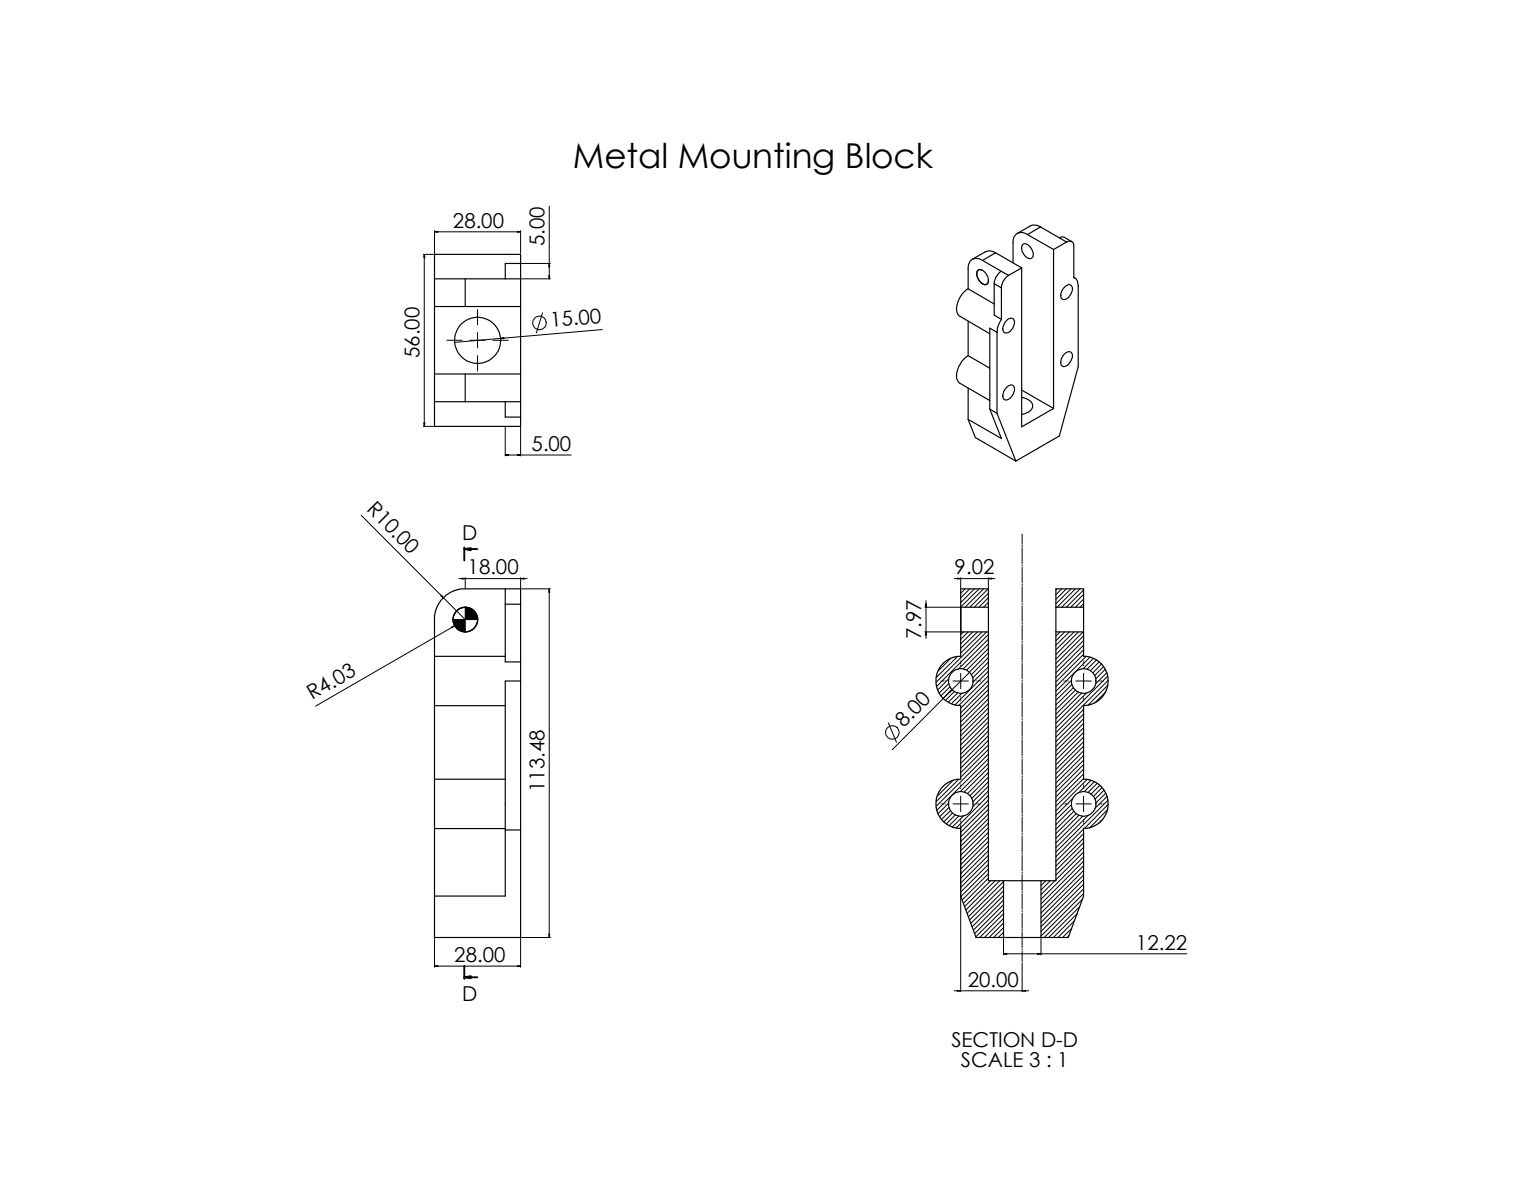
ISO-10303-21;
HEADER;
FILE_DESCRIPTION (('STEP AP214'),
    '1' );
FILE_NAME ('Metal Mounting Block.step',
    '2026-10-20T14:49:59',
    ( '' ),
    ( '' ),
    'SwSTEP 2.0',
    'SolidWorks 2025',
    '' );
FILE_SCHEMA (( 'AUTOMOTIVE_DESIGN' ));
ENDSEC;

DATA;
#3=LINE ( 'NONE', #5660, #7079 ) ;
#10=FACE_BOUND ( 'NONE', #10352, .T. ) ;
#13=VERTEX_POINT ( 'NONE', #5217 ) ;
#17=EDGE_CURVE ( 'NONE', #7054, #8863, #10257, .T. ) ;
#35=DIRECTION ( 'NONE',  ( 1.000000000000000000, -0.000000000000000000, -0.000000000000000000 ) ) ;
#39=VERTEX_POINT ( 'NONE', #5423 ) ;
#41=CARTESIAN_POINT ( 'NONE',  ( -7.293506896408097795, 145.5696653505793563, -20.00000000000000711 ) ) ;
#51=CYLINDRICAL_SURFACE ( 'NONE', #8825, 4.000000000000000000 ) ;
#52=AXIS2_PLACEMENT_3D ( 'NONE', #3037, #3895, #4040 ) ;
#61=AXIS2_PLACEMENT_3D ( 'NONE', #1587, #8044, #3822 ) ;
#66=LINE ( 'NONE', #8964, #2259 ) ;
#67=DIRECTION ( 'NONE',  ( -0.7071067811864983899, 8.659560562354331352E-17, 0.7071067811865966446 ) ) ;
#72=ORIENTED_EDGE ( 'NONE', *, *, #1454, .F. ) ;
#89=ADVANCED_FACE ( 'NONE', ( #9520 ), #9630, .T. ) ;
#91=DIRECTION ( 'NONE',  ( 0.000000000000000000, -1.222897680782651471E-16, 1.000000000000000000 ) ) ;
#95=DIRECTION ( 'NONE',  ( -0.000000000000000000, -0.000000000000000000, 1.000000000000000000 ) ) ;
#97=EDGE_LOOP ( 'NONE', ( #5379, #7947, #3762, #7012 ) ) ;
#99=ORIENTED_EDGE ( 'NONE', *, *, #5544, .F. ) ;
#104=VECTOR ( 'NONE', #4491, 1000.000000000000000 ) ;
#113=VECTOR ( 'NONE', #5634, 1000.000000000000000 ) ;
#121=VECTOR ( 'NONE', #5228, 1000.000000000000000 ) ;
#124=CIRCLE ( 'NONE', #1803, 7.500000000000000000 ) ;
#131=ORIENTED_EDGE ( 'NONE', *, *, #6804, .F. ) ;
#138=CARTESIAN_POINT ( 'NONE',  ( -7.293506896408097795, 50.54838324668256888, 20.00000000000001776 ) ) ;
#152=FACE_OUTER_BOUND ( 'NONE', #4686, .T. ) ;
#153=DIRECTION ( 'NONE',  ( -1.000000000000000000, 0.000000000000000000, 0.000000000000000000 ) ) ;
#156=ORIENTED_EDGE ( 'NONE', *, *, #9691, .F. ) ;
#157=CARTESIAN_POINT ( 'NONE',  ( -2.293506896408097795, 120.5696653505793705, 20.00000000000000711 ) ) ;
#167=ORIENTED_EDGE ( 'NONE', *, *, #1641, .F. ) ;
#188=CARTESIAN_POINT ( 'NONE',  ( -30.29350689640809335, 37.08684478514406635, 0.000000000000000000 ) ) ;
#190=CARTESIAN_POINT ( 'NONE',  ( -7.293506896408097795, 50.54838324668256888, -20.00000000000001776 ) ) ;
#195=VERTEX_POINT ( 'NONE', #3902 ) ;
#200=DIRECTION ( 'NONE',  ( 0.000000000000000000, 1.000000000000000000, 0.000000000000000000 ) ) ;
#203=EDGE_LOOP ( 'NONE', ( #8240, #8305, #10001, #6976, #3187, #9611 ) ) ;
#209=FACE_OUTER_BOUND ( 'NONE', #8382, .T. ) ;
#224=CARTESIAN_POINT ( 'NONE',  ( -30.29350689640809335, 80.56966535057935630, -24.00000000000000711 ) ) ;
#255=AXIS2_PLACEMENT_3D ( 'NONE', #5974, #6135, #9270 ) ;
#270=LINE ( 'NONE', #5923, #8481 ) ;
#272=ORIENTED_EDGE ( 'NONE', *, *, #9010, .T. ) ;
#279=FACE_OUTER_BOUND ( 'NONE', #7883, .T. ) ;
#283=EDGE_LOOP ( 'NONE', ( #4736, #4335, #5874, #8256, #8188 ) ) ;
#288=VERTEX_POINT ( 'NONE', #1021 ) ;
#295=VECTOR ( 'NONE', #753, 1000.000000000000114 ) ;
#302=EDGE_CURVE ( 'NONE', #5556, #3604, #5045, .T. ) ;
#303=EDGE_CURVE ( 'NONE', #4587, #5189, #10304, .T. ) ;
#316=VECTOR ( 'NONE', #2440, 1000.000000000000000 ) ;
#317=EDGE_CURVE ( 'NONE', #10264, #2451, #2832, .T. ) ;
#339=ORIENTED_EDGE ( 'NONE', *, *, #9708, .F. ) ;
#344=DIRECTION ( 'NONE',  ( 1.000000000000000000, -0.000000000000000000, -0.000000000000000000 ) ) ;
#353=CYLINDRICAL_SURFACE ( 'NONE', #7185, 4.000000000000000000 ) ;
#355=CYLINDRICAL_SURFACE ( 'NONE', #5843, 4.000000000000000000 ) ;
#356=EDGE_CURVE ( 'NONE', #5466, #9263, #915, .T. ) ;
#372=CARTESIAN_POINT ( 'NONE',  ( -20.29350689640809691, 140.5696653505793563, 20.00000000000002132 ) ) ;
#376=AXIS2_PLACEMENT_3D ( 'NONE', #9836, #6639, #8122 ) ;
#383=ORIENTED_EDGE ( 'NONE', *, *, #664, .T. ) ;
#398=DIRECTION ( 'NONE',  ( 1.000000000000000000, -0.000000000000000000, -0.000000000000000000 ) ) ;
#410=EDGE_LOOP ( 'NONE', ( #1681, #5239, #2854, #5762 ) ) ;
#418=CARTESIAN_POINT ( 'NONE',  ( -7.293506896408097795, 4.007378841484243628E-15, -28.00000000000002132 ) ) ;
#419=ORIENTED_EDGE ( 'NONE', *, *, #2627, .T. ) ;
#432=DIRECTION ( 'NONE',  ( 1.000000000000000000, -0.000000000000000000, -0.000000000000000000 ) ) ;
#438=ORIENTED_EDGE ( 'NONE', *, *, #7577, .T. ) ;
#443=ORIENTED_EDGE ( 'NONE', *, *, #6054, .F. ) ;
#450=ORIENTED_EDGE ( 'NONE', *, *, #5738, .F. ) ;
#452=VECTOR ( 'NONE', #3941, 1000.000000000000000 ) ;
#458=DIRECTION ( 'NONE',  ( 0.000000000000000000, 0.000000000000000000, 1.000000000000000000 ) ) ;
#467=VECTOR ( 'NONE', #4578, 1000.000000000000114 ) ;
#469=DIRECTION ( 'NONE',  ( 1.000000000000000000, 0.000000000000000000, 0.000000000000000000 ) ) ;
#476=VECTOR ( 'NONE', #3446, 1000.000000000000000 ) ;
#484=DIRECTION ( 'NONE',  ( 0.000000000000000000, -1.000000000000000000, 1.222897680782651471E-16 ) ) ;
#489=ADVANCED_FACE ( 'NONE', ( #10089 ), #9183, .T. ) ;
#495=DIRECTION ( 'NONE',  ( 0.000000000000000000, -1.000000000000000000, -1.222897680782651224E-16 ) ) ;
#504=DIRECTION ( 'NONE',  ( 1.000000000000000000, 0.000000000000000000, 0.000000000000000000 ) ) ;
#510=VERTEX_POINT ( 'NONE', #5251 ) ;
#512=ORIENTED_EDGE ( 'NONE', *, *, #1198, .F. ) ;
#522=DIRECTION ( 'NONE',  ( -1.000000000000000000, -0.000000000000000000, -0.000000000000000000 ) ) ;
#524=CARTESIAN_POINT ( 'NONE',  ( -30.29350689640809335, 140.5696653505793563, -20.00000000000000355 ) ) ;
#544=CARTESIAN_POINT ( 'NONE',  ( -30.29350689640809335, 37.08684478514406635, -15.00000000000000355 ) ) ;
#545=ADVANCED_FACE ( 'NONE', ( #7912, #2343, #6211, #4819, #2293 ), #3832, .F. ) ;
#567=ORIENTED_EDGE ( 'NONE', *, *, #7866, .T. ) ;
#579=CARTESIAN_POINT ( 'NONE',  ( -20.29350689640809691, 140.5696653505793563, -20.00000000000000355 ) ) ;
#582=CIRCLE ( 'NONE', #8191, 5.000000000000000888 ) ;
#592=ORIENTED_EDGE ( 'NONE', *, *, #303, .F. ) ;
#596=VERTEX_POINT ( 'NONE', #7217 ) ;
#603=ORIENTED_EDGE ( 'NONE', *, *, #3823, .F. ) ;
#621=CARTESIAN_POINT ( 'NONE',  ( -30.29350689640809335, 145.5696653505793563, 20.00000000000000711 ) ) ;
#633=DIRECTION ( 'NONE',  ( 0.000000000000000000, -1.000000000000000000, 0.000000000000000000 ) ) ;
#634=EDGE_CURVE ( 'NONE', #2019, #13, #4708, .T. ) ;
#656=PLANE ( 'NONE',  #8662 ) ;
#657=CARTESIAN_POINT ( 'NONE',  ( -7.293506896408097795, 4.007378841484243628E-15, 28.00000000000002132 ) ) ;
#658=CARTESIAN_POINT ( 'NONE',  ( -7.293506896408097795, 80.56966535057935630, -20.00000000000000711 ) ) ;
#660=CIRCLE ( 'NONE', #4540, 4.000000000000000000 ) ;
#664=EDGE_CURVE ( 'NONE', #954, #4361, #955, .T. ) ;
#667=DIRECTION ( 'NONE',  ( 0.000000000000000000, 0.000000000000000000, 1.000000000000000000 ) ) ;
#675=EDGE_LOOP ( 'NONE', ( #1333, #9999, #2381, #686 ) ) ;
#676=ADVANCED_FACE ( 'NONE', ( #10, #4242 ), #5668, .F. ) ;
#686=ORIENTED_EDGE ( 'NONE', *, *, #10087, .F. ) ;
#716=VERTEX_POINT ( 'NONE', #2543 ) ;
#731=EDGE_CURVE ( 'NONE', #8244, #5058, #3289, .T. ) ;
#734=CIRCLE ( 'NONE', #7849, 4.000000000000000000 ) ;
#737=DIRECTION ( 'NONE',  ( 0.000000000000000000, 0.000000000000000000, 1.000000000000000000 ) ) ;
#740=CARTESIAN_POINT ( 'NONE',  ( -7.293506896408097795, 145.5696653505793563, -25.00000000000000711 ) ) ;
#750=AXIS2_PLACEMENT_3D ( 'NONE', #8663, #6275, #5427 ) ;
#753=DIRECTION ( 'NONE',  ( 0.000000000000000000, -0.9374252720097652203, -0.3481865296036273372 ) ) ;
#761=CARTESIAN_POINT ( 'NONE',  ( -7.293506896408097795, 80.56966535057935630, 20.00000000000000711 ) ) ;
#763=AXIS2_PLACEMENT_3D ( 'NONE', #4850, #200, #3320 ) ;
#767=DIRECTION ( 'NONE',  ( -1.000000000000000000, 0.000000000000000000, 0.000000000000000000 ) ) ;
#777=LINE ( 'NONE', #4799, #5594 ) ;
#780=VECTOR ( 'NONE', #9895, 1000.000000000000000 ) ;
#781=EDGE_LOOP ( 'NONE', ( #592, #10254 ) ) ;
#782=DIRECTION ( 'NONE',  ( 1.000000000000000000, -0.000000000000000000, -0.000000000000000000 ) ) ;
#793=CIRCLE ( 'NONE', #2484, 3.999999999999989786 ) ;
#801=DIRECTION ( 'NONE',  ( 0.000000000000000000, -1.000000000000000000, -1.222897680782651471E-16 ) ) ;
#812=ORIENTED_EDGE ( 'NONE', *, *, #634, .T. ) ;
#822=VERTEX_POINT ( 'NONE', #4455 ) ;
#827=DIRECTION ( 'NONE',  ( 0.000000000000000000, 0.000000000000000000, 1.000000000000000000 ) ) ;
#832=VECTOR ( 'NONE', #8468, 1000.000000000000000 ) ;
#843=ORIENTED_EDGE ( 'NONE', *, *, #5371, .T. ) ;
#846=EDGE_CURVE ( 'NONE', #10164, #6362, #660, .T. ) ;
#848=DIRECTION ( 'NONE',  ( 1.000000000000000000, 0.000000000000000000, -0.000000000000000000 ) ) ;
#850=DIRECTION ( 'NONE',  ( 0.000000000000000000, -1.734723475976808278E-15, 1.000000000000000000 ) ) ;
#852=VERTEX_POINT ( 'NONE', #2061 ) ;
#855=DIRECTION ( 'NONE',  ( 0.000000000000000000, -0.9374252720097652203, 0.3481865296036273372 ) ) ;
#856=EDGE_CURVE ( 'NONE', #6933, #6085, #6838, .T. ) ;
#859=AXIS2_PLACEMENT_3D ( 'NONE', #9746, #8298, #5696 ) ;
#860=CARTESIAN_POINT ( 'NONE',  ( -20.29350689640809691, 150.5696653505793563, 20.00000000000000355 ) ) ;
#861=DIRECTION ( 'NONE',  ( 0.000000000000000000, -1.000000000000000000, -1.222897680782651224E-16 ) ) ;
#875=ORIENTED_EDGE ( 'NONE', *, *, #5133, .T. ) ;
#878=DIRECTION ( 'NONE',  ( 0.000000000000000000, -1.000000000000000000, 0.000000000000000000 ) ) ;
#885=CARTESIAN_POINT ( 'NONE',  ( -30.29350689640809335, -0.3998014571812398832, 1.076388538564875708 ) ) ;
#904=DIRECTION ( 'NONE',  ( 1.000000000000000000, -0.000000000000000000, -0.000000000000000000 ) ) ;
#911=DIRECTION ( 'NONE',  ( 0.000000000000000000, 0.000000000000000000, 1.000000000000000000 ) ) ;
#915=LINE ( 'NONE', #4150, #9967 ) ;
#931=CARTESIAN_POINT ( 'NONE',  ( -16.29350689640809691, -19.43033464942062238, 0.000000000000000000 ) ) ;
#935=CARTESIAN_POINT ( 'NONE',  ( -20.29350689640809691, 140.5696653505793563, -20.00000000000000711 ) ) ;
#938=DIRECTION ( 'NONE',  ( 1.000000000000000000, -0.000000000000000000, -0.000000000000000000 ) ) ;
#941=VERTEX_POINT ( 'NONE', #3973 ) ;
#942=DIRECTION ( 'NONE',  ( -1.000000000000000000, -0.000000000000000000, -0.000000000000000000 ) ) ;
#945=LINE ( 'NONE', #2479, #10150 ) ;
#946=DIRECTION ( 'NONE',  ( 0.000000000000000000, -0.9374252720097652203, 0.3481865296036273372 ) ) ;
#952=ORIENTED_EDGE ( 'NONE', *, *, #17, .F. ) ;
#954=VERTEX_POINT ( 'NONE', #10390 ) ;
#955=LINE ( 'NONE', #8910, #476 ) ;
#966=ORIENTED_EDGE ( 'NONE', *, *, #993, .T. ) ;
#992=DIRECTION ( 'NONE',  ( -1.000000000000000000, 0.000000000000000000, 0.000000000000000000 ) ) ;
#993=EDGE_CURVE ( 'NONE', #2923, #9336, #1538, .T. ) ;
#1003=( GEOMETRIC_REPRESENTATION_CONTEXT ( 3 ) GLOBAL_UNCERTAINTY_ASSIGNED_CONTEXT ( ( #1512 ) ) GLOBAL_UNIT_ASSIGNED_CONTEXT ( ( #2813, #9988, #8280 ) ) REPRESENTATION_CONTEXT ( 'NONE', 'WORKASPACE' ) );
#1006=EDGE_CURVE ( 'NONE', #6072, #6663, #8634, .T. ) ;
#1015=LINE ( 'NONE', #524, #8409 ) ;
#1020=PRODUCT_DEFINITION_CONTEXT ( 'detailed design', #8151, 'design' ) ;
#1021=CARTESIAN_POINT ( 'NONE',  ( -16.29350689640810756, 140.5696653505793563, -10.98204862120179648 ) ) ;
#1034=VECTOR ( 'NONE', #1710, 1000.000000000000000 ) ;
#1036=FACE_OUTER_BOUND ( 'NONE', #9629, .T. ) ;
#1043=VERTEX_POINT ( 'NONE', #1377 ) ;
#1049=VECTOR ( 'NONE', #861, 1000.000000000000000 ) ;
#1060=LINE ( 'NONE', #6623, #5109 ) ;
#1069=ORIENTED_EDGE ( 'NONE', *, *, #8198, .T. ) ;
#1071=ORIENTED_EDGE ( 'NONE', *, *, #664, .F. ) ;
#1074=LINE ( 'NONE', #1819, #4670 ) ;
#1079=VERTEX_POINT ( 'NONE', #5656 ) ;
#1080=LINE ( 'NONE', #1926, #7329 ) ;
#1083=VERTEX_POINT ( 'NONE', #8893 ) ;
#1088=DIRECTION ( 'NONE',  ( 1.000000000000000000, -0.000000000000000000, -0.000000000000000000 ) ) ;
#1100=ORIENTED_EDGE ( 'NONE', *, *, #4696, .T. ) ;
#1101=CARTESIAN_POINT ( 'NONE',  ( -2.293506896408097795, 145.5696653505793563, -25.00000000000000711 ) ) ;
#1102=DIRECTION ( 'NONE',  ( 1.000000000000000000, 0.000000000000000000, 0.000000000000000000 ) ) ;
#1105=CARTESIAN_POINT ( 'NONE',  ( -20.29350689640809691, 140.5696653505793563, 0.000000000000000000 ) ) ;
#1109=ORIENTED_EDGE ( 'NONE', *, *, #3823, .T. ) ;
#1111=DIRECTION ( 'NONE',  ( -1.000000000000000000, 0.000000000000000000, 0.000000000000000000 ) ) ;
#1116=LINE ( 'NONE', #7323, #6386 ) ;
#1117=VERTEX_POINT ( 'NONE', #7257 ) ;
#1131=CIRCLE ( 'NONE', #7064, 10.00000000000000888 ) ;
#1140=EDGE_CURVE ( 'NONE', #10264, #9816, #2426, .T. ) ;
#1142=CARTESIAN_POINT ( 'NONE',  ( -30.29350689640809335, 80.56966535057935630, 20.00000000000000711 ) ) ;
#1146=EDGE_LOOP ( 'NONE', ( #812, #8947 ) ) ;
#1148=CARTESIAN_POINT ( 'NONE',  ( -20.29350689640809691, 140.5696653505793563, 20.00000000000000355 ) ) ;
#1152=CIRCLE ( 'NONE', #3873, 4.000000000000000000 ) ;
#1157=CARTESIAN_POINT ( 'NONE',  ( -30.29350689640809335, 37.08684478514406635, 15.00000000000000355 ) ) ;
#1160=FACE_OUTER_BOUND ( 'NONE', #2223, .T. ) ;
#1161=VECTOR ( 'NONE', #7788, 1000.000000000000000 ) ;
#1167=ORIENTED_EDGE ( 'NONE', *, *, #8133, .T. ) ;
#1175=EDGE_LOOP ( 'NONE', ( #6473, #7794, #10471, #9288 ) ) ;
#1183=DIRECTION ( 'NONE',  ( -1.000000000000000000, 0.000000000000000000, 0.000000000000000000 ) ) ;
#1190=DIRECTION ( 'NONE',  ( 0.000000000000000000, 0.000000000000000000, 1.000000000000000000 ) ) ;
#1193=FACE_OUTER_BOUND ( 'NONE', #1279, .T. ) ;
#1196=ORIENTED_EDGE ( 'NONE', *, *, #1532, .F. ) ;
#1198=EDGE_CURVE ( 'NONE', #5466, #7089, #3190, .T. ) ;
#1199=EDGE_CURVE ( 'NONE', #5863, #1913, #1792, .T. ) ;
#1205=ORIENTED_EDGE ( 'NONE', *, *, #2933, .T. ) ;
#1206=DIRECTION ( 'NONE',  ( 0.000000000000000000, -1.000000000000000000, -1.222897680782651224E-16 ) ) ;
#1220=EDGE_CURVE ( 'NONE', #4525, #2500, #3708, .T. ) ;
#1225=CARTESIAN_POINT ( 'NONE',  ( -2.293506896408097795, 150.5696653505793563, 20.00000000000000711 ) ) ;
#1234=DIRECTION ( 'NONE',  ( 0.000000000000000000, -1.431206729101514631E-16, 1.000000000000000000 ) ) ;
#1247=VECTOR ( 'NONE', #1264, 1000.000000000000000 ) ;
#1249=ORIENTED_EDGE ( 'NONE', *, *, #7540, .T. ) ;
#1258=LINE ( 'NONE', #2847, #104 ) ;
#1264=DIRECTION ( 'NONE',  ( 1.000000000000000000, -0.000000000000000000, -0.000000000000000000 ) ) ;
#1265=PLANE ( 'NONE',  #6164 ) ;
#1268=EDGE_LOOP ( 'NONE', ( #3343, #2802, #567, #512, #4602, #10138, #10269 ) ) ;
#1276=DIRECTION ( 'NONE',  ( 1.000000000000000000, -0.000000000000000000, -0.000000000000000000 ) ) ;
#1279=EDGE_LOOP ( 'NONE', ( #3702, #9720, #2445, #3175 ) ) ;
#1282=VERTEX_POINT ( 'NONE', #9970 ) ;
#1291=EDGE_LOOP ( 'NONE', ( #7966, #7553 ) ) ;
#1295=ORIENTED_EDGE ( 'NONE', *, *, #7737, .F. ) ;
#1302=DIRECTION ( 'NONE',  ( 1.000000000000000000, -0.000000000000000000, -0.000000000000000000 ) ) ;
#1311=ORIENTED_EDGE ( 'NONE', *, *, #2487, .F. ) ;
#1312=LINE ( 'NONE', #7938, #10266 ) ;
#1315=CARTESIAN_POINT ( 'NONE',  ( -30.29350689640809335, 120.5696653505793705, -20.00000000000000711 ) ) ;
#1318=FACE_OUTER_BOUND ( 'NONE', #283, .T. ) ;
#1322=EDGE_CURVE ( 'NONE', #10164, #4525, #1258, .T. ) ;
#1331=DIRECTION ( 'NONE',  ( 0.000000000000000000, 0.000000000000000000, 1.000000000000000000 ) ) ;
#1333=ORIENTED_EDGE ( 'NONE', *, *, #9472, .T. ) ;
#1334=ORIENTED_EDGE ( 'NONE', *, *, #1987, .T. ) ;
#1339=ORIENTED_EDGE ( 'NONE', *, *, #1006, .F. ) ;
#1340=VECTOR ( 'NONE', #10000, 1000.000000000000000 ) ;
#1344=CYLINDRICAL_SURFACE ( 'NONE', #2810, 3.999999999999989786 ) ;
#1352=VERTEX_POINT ( 'NONE', #8306 ) ;
#1353=EDGE_CURVE ( 'NONE', #9176, #941, #4338, .T. ) ;
#1354=CARTESIAN_POINT ( 'NONE',  ( -7.293506896408097795, 126.8146633489777599, 25.00000000000000355 ) ) ;
#1359=VERTEX_POINT ( 'NONE', #1101 ) ;
#1367=EDGE_LOOP ( 'NONE', ( #7375, #167, #6674, #5877 ) ) ;
#1370=CARTESIAN_POINT ( 'NONE',  ( -16.26850689640809478, 140.5696653505793563, 20.00000000000002132 ) ) ;
#1377=CARTESIAN_POINT ( 'NONE',  ( -16.29350689640809691, 55.56966535057936341, -7.500000000000000000 ) ) ;
#1380=EDGE_CURVE ( 'NONE', #8244, #9480, #7671, .T. ) ;
#1403=VERTEX_POINT ( 'NONE', #3862 ) ;
#1405=CIRCLE ( 'NONE', #52, 5.000000000000000888 ) ;
#1407=ADVANCED_FACE ( 'NONE', ( #3750 ), #2157, .T. ) ;
#1418=ORIENTED_EDGE ( 'NONE', *, *, #9964, .T. ) ;
#1419=DIRECTION ( 'NONE',  ( 1.000000000000000000, 0.000000000000000000, 0.000000000000000000 ) ) ;
#1439=VERTEX_POINT ( 'NONE', #8785 ) ;
#1442=ORIENTED_EDGE ( 'NONE', *, *, #5543, .T. ) ;
#1454=EDGE_CURVE ( 'NONE', #5461, #6490, #1312, .T. ) ;
#1468=ADVANCED_FACE ( 'NONE', ( #1526 ), #3056, .T. ) ;
#1471=DIRECTION ( 'NONE',  ( -1.000000000000000000, 0.000000000000000000, 0.000000000000000000 ) ) ;
#1481=DIRECTION ( 'NONE',  ( -0.000000000000000000, 1.222897680782651471E-16, -1.000000000000000000 ) ) ;
#1485=VECTOR ( 'NONE', #3097, 1000.000000000000000 ) ;
#1501=AXIS2_PLACEMENT_3D ( 'NONE', #5590, #8724, #1471 ) ;
#1512=UNCERTAINTY_MEASURE_WITH_UNIT (LENGTH_MEASURE( 1.000000000000000082E-05 ), #2813, 'distance_accuracy_value', 'NONE');
#1516=EDGE_CURVE ( 'NONE', #2007, #1282, #9590, .T. ) ;
#1526=FACE_OUTER_BOUND ( 'NONE', #1367, .T. ) ;
#1532=EDGE_CURVE ( 'NONE', #9083, #1931, #1954, .T. ) ;
#1537=ORIENTED_EDGE ( 'NONE', *, *, #7658, .T. ) ;
#1538=LINE ( 'NONE', #5561, #7759 ) ;
#1541=LINE ( 'NONE', #3975, #3278 ) ;
#1546=VECTOR ( 'NONE', #3114, 1000.000000000000000 ) ;
#1552=AXIS2_PLACEMENT_3D ( 'NONE', #7863, #7967, #10359 ) ;
#1556=ORIENTED_EDGE ( 'NONE', *, *, #6748, .F. ) ;
#1571=ORIENTED_EDGE ( 'NONE', *, *, #634, .F. ) ;
#1587=CARTESIAN_POINT ( 'NONE',  ( -30.29350689640809335, 80.56966535057935630, -20.00000000000000711 ) ) ;
#1593=ORIENTED_EDGE ( 'NONE', *, *, #4957, .F. ) ;
#1594=EDGE_CURVE ( 'NONE', #5925, #3441, #1074, .T. ) ;
#1596=LINE ( 'NONE', #8757, #5448 ) ;
#1597=AXIS2_PLACEMENT_3D ( 'NONE', #5049, #7006, #484 ) ;
#1624=CARTESIAN_POINT ( 'NONE',  ( -7.293506896408097795, -3.651280424770854409E-15, 24.99999999999998579 ) ) ;
#1632=EDGE_LOOP ( 'NONE', ( #2607, #2789, #4830, #9276, #8779, #2786, #443, #7436, #10424, #10141, #9748, #952, #4956, #10358, #2505, #2868, #10031, #8560, #156, #3347 ) ) ;
#1633=DIRECTION ( 'NONE',  ( 0.000000000000000000, 0.000000000000000000, 1.000000000000000000 ) ) ;
#1637=LINE ( 'NONE', #1796, #4788 ) ;
#1641=EDGE_CURVE ( 'NONE', #1403, #5730, #6745, .T. ) ;
#1653=ORIENTED_EDGE ( 'NONE', *, *, #1641, .T. ) ;
#1654=ADVANCED_FACE ( 'NONE', ( #1920 ), #3363, .F. ) ;
#1668=LINE ( 'NONE', #188, #113 ) ;
#1669=EDGE_CURVE ( 'NONE', #2192, #195, #5789, .T. ) ;
#1676=DIRECTION ( 'NONE',  ( -1.000000000000000000, 0.000000000000000000, 0.000000000000000000 ) ) ;
#1681=ORIENTED_EDGE ( 'NONE', *, *, #846, .T. ) ;
#1682=DIRECTION ( 'NONE',  ( -1.000000000000000000, 0.000000000000000000, 0.000000000000000000 ) ) ;
#1683=EDGE_CURVE ( 'NONE', #1083, #1913, #4521, .T. ) ;
#1686=DIRECTION ( 'NONE',  ( 0.000000000000000000, 1.000000000000000000, -1.460512169908342690E-16 ) ) ;
#1691=CARTESIAN_POINT ( 'NONE',  ( -7.293506896408105789, 150.5696653505793563, -20.00000000000000355 ) ) ;
#1695=VERTEX_POINT ( 'NONE', #7756 ) ;
#1706=CIRCLE ( 'NONE', #8135, 7.999999999999991118 ) ;
#1710=DIRECTION ( 'NONE',  ( -0.000000000000000000, -0.000000000000000000, 1.000000000000000000 ) ) ;
#1719=VECTOR ( 'NONE', #6591, 1000.000000000000000 ) ;
#1728=DIRECTION ( 'NONE',  ( -1.000000000000000000, 0.000000000000000000, 0.000000000000000000 ) ) ;
#1734=AXIS2_PLACEMENT_3D ( 'NONE', #8821, #10265, #8024 ) ;
#1736=CARTESIAN_POINT ( 'NONE',  ( -30.29350689640809335, -0.3998014571812398832, -1.076388538564875708 ) ) ;
#1744=CARTESIAN_POINT ( 'NONE',  ( -20.29350689640810401, 150.5696653505793563, -10.98204862120179826 ) ) ;
#1748=AXIS2_PLACEMENT_3D ( 'NONE', #3396, #6681, #1860 ) ;
#1762=UNCERTAINTY_MEASURE_WITH_UNIT (LENGTH_MEASURE( 1.000000000000000082E-05 ), #9279, 'distance_accuracy_value', 'NONE');
#1772=EDGE_CURVE ( 'NONE', #510, #4261, #8231, .T. ) ;
#1773=ADVANCED_FACE ( 'NONE', ( #8650 ), #1344, .F. ) ;
#1776=ORIENTED_EDGE ( 'NONE', *, *, #6748, .T. ) ;
#1784=FACE_OUTER_BOUND ( 'NONE', #6548, .T. ) ;
#1786=EDGE_CURVE ( 'NONE', #954, #9488, #2649, .T. ) ;
#1788=EDGE_LOOP ( 'NONE', ( #8956, #7525, #5665, #603 ) ) ;
#1792=LINE ( 'NONE', #4859, #8780 ) ;
#1793=CARTESIAN_POINT ( 'NONE',  ( -7.293506896408097795, -3.651280424770854409E-15, -24.99999999999998579 ) ) ;
#1796=CARTESIAN_POINT ( 'NONE',  ( -7.293506896408097795, 72.08684478514406635, 28.00000000000001066 ) ) ;
#1803=AXIS2_PLACEMENT_3D ( 'NONE', #5143, #9067, #3562 ) ;
#1804=ORIENTED_EDGE ( 'NONE', *, *, #7866, .F. ) ;
#1814=AXIS2_PLACEMENT_3D ( 'NONE', #1142, #1088, #6757 ) ;
#1819=CARTESIAN_POINT ( 'NONE',  ( -7.293506896408097795, 2.445795361565304815E-15, -20.00000000000002132 ) ) ;
#1831=EDGE_CURVE ( 'NONE', #4261, #596, #7858, .T. ) ;
#1837=AXIS2_PLACEMENT_3D ( 'NONE', #5705, #6667, #1633 ) ;
#1838=ORIENTED_EDGE ( 'NONE', *, *, #2430, .T. ) ;
#1844=CARTESIAN_POINT ( 'NONE',  ( -30.29350689640809335, 50.54838324668256888, 20.00000000000001776 ) ) ;
#1845=ADVANCED_FACE ( 'NONE', ( #4726 ), #8704, .F. ) ;
#1860=DIRECTION ( 'NONE',  ( 0.000000000000000000, 0.000000000000000000, 1.000000000000000000 ) ) ;
#1861=CYLINDRICAL_SURFACE ( 'NONE', #8080, 4.000000000000000000 ) ;
#1870=CARTESIAN_POINT ( 'NONE',  ( -2.293506896408097795, 145.5696653505793563, 20.00000000000000711 ) ) ;
#1871=CARTESIAN_POINT ( 'NONE',  ( -24.29350689640808980, 140.5696653505793563, 19.97500000000000853 ) ) ;
#1888=EDGE_CURVE ( 'NONE', #822, #7959, #6023, .T. ) ;
#1891=ORIENTED_EDGE ( 'NONE', *, *, #856, .T. ) ;
#1894=DIRECTION ( 'NONE',  ( -1.000000000000000000, 0.000000000000000000, 0.000000000000000000 ) ) ;
#1897=VECTOR ( 'NONE', #9971, 1000.000000000000000 ) ;
#1898=DIRECTION ( 'NONE',  ( 1.000000000000000000, 0.000000000000000000, 0.000000000000000000 ) ) ;
#1911=FACE_OUTER_BOUND ( 'NONE', #1175, .T. ) ;
#1913=VERTEX_POINT ( 'NONE', #7172 ) ;
#1920=FACE_OUTER_BOUND ( 'NONE', #3172, .T. ) ;
#1926=CARTESIAN_POINT ( 'NONE',  ( -30.29350689640809335, 120.5696653505793705, 16.00000000000000711 ) ) ;
#1931=VERTEX_POINT ( 'NONE', #5291 ) ;
#1937=DIRECTION ( 'NONE',  ( 0.000000000000000000, 0.000000000000000000, 1.000000000000000000 ) ) ;
#1942=PLANE ( 'NONE',  #7568 ) ;
#1948=DIRECTION ( 'NONE',  ( 1.000000000000000000, -0.000000000000000000, -0.000000000000000000 ) ) ;
#1954=CIRCLE ( 'NONE', #8733, 3.999999999999989786 ) ;
#1956=( NAMED_UNIT ( * ) PLANE_ANGLE_UNIT ( ) SI_UNIT ( $, .RADIAN. ) );
#1971=DIRECTION ( 'NONE',  ( -1.000000000000000000, 0.000000000000000000, 0.000000000000000000 ) ) ;
#1981=AXIS2_PLACEMENT_3D ( 'NONE', #1736, #2735, #4229 ) ;
#1983=DIRECTION ( 'NONE',  ( 1.000000000000000000, -0.000000000000000000, -0.000000000000000000 ) ) ;
#1987=EDGE_CURVE ( 'NONE', #5429, #6933, #4007, .T. ) ;
#1993=CARTESIAN_POINT ( 'NONE',  ( -30.29350689640809335, 128.5696653505793847, 20.00000000000000711 ) ) ;
#1998=LINE ( 'NONE', #7037, #7228 ) ;
#2004=DIRECTION ( 'NONE',  ( -1.000000000000000000, 0.000000000000000000, 0.000000000000000000 ) ) ;
#2007=VERTEX_POINT ( 'NONE', #10178 ) ;
#2019=VERTEX_POINT ( 'NONE', #2910 ) ;
#2026=DIRECTION ( 'NONE',  ( 0.000000000000000000, 1.000000000000000000, 1.460512169908342690E-16 ) ) ;
#2027=DIRECTION ( 'NONE',  ( -1.000000000000000000, 0.000000000000000000, 0.000000000000000000 ) ) ;
#2035=CARTESIAN_POINT ( 'NONE',  ( -30.29350689640809335, -0.3998014571812398832, 1.076388538564875708 ) ) ;
#2043=ORIENTED_EDGE ( 'NONE', *, *, #1322, .T. ) ;
#2055=CIRCLE ( 'NONE', #9857, 7.999999999999991118 ) ;
#2058=ORIENTED_EDGE ( 'NONE', *, *, #1831, .F. ) ;
#2061=CARTESIAN_POINT ( 'NONE',  ( -30.29350689640809335, 140.5696653505793563, -20.00000000000000355 ) ) ;
#2062=LINE ( 'NONE', #4456, #8497 ) ;
#2067=CARTESIAN_POINT ( 'NONE',  ( -30.29350689640809335, 120.5696653505793705, 20.00000000000000711 ) ) ;
#2097=ORIENTED_EDGE ( 'NONE', *, *, #3900, .F. ) ;
#2103=DIRECTION ( 'NONE',  ( 0.000000000000000000, 0.000000000000000000, 1.000000000000000000 ) ) ;
#2107=LINE ( 'NONE', #10065, #4468 ) ;
#2109=ADVANCED_FACE ( 'NONE', ( #4712 ), #8093, .T. ) ;
#2116=AXIS2_PLACEMENT_3D ( 'NONE', #8691, #10346, #3824 ) ;
#2121=EDGE_CURVE ( 'NONE', #6484, #6663, #2373, .T. ) ;
#2125=EDGE_CURVE ( 'NONE', #9816, #288, #793, .T. ) ;
#2127=ORIENTED_EDGE ( 'NONE', *, *, #5471, .T. ) ;
#2145=CIRCLE ( 'NONE', #2819, 4.000000000000000000 ) ;
#2149=ORIENTED_EDGE ( 'NONE', *, *, #7672, .F. ) ;
#2157=CYLINDRICAL_SURFACE ( 'NONE', #3488, 5.000000000000000888 ) ;
#2158=LINE ( 'NONE', #8124, #1049 ) ;
#2173=ORIENTED_EDGE ( 'NONE', *, *, #8842, .T. ) ;
#2180=AXIS2_PLACEMENT_3D ( 'NONE', #5276, #767, #7880 ) ;
#2189=DIRECTION ( 'NONE',  ( 0.000000000000000000, 0.000000000000000000, 1.000000000000000000 ) ) ;
#2192=VERTEX_POINT ( 'NONE', #8040 ) ;
#2201=DIRECTION ( 'NONE',  ( -1.000000000000000000, 0.000000000000000000, 0.000000000000000000 ) ) ;
#2206=EDGE_LOOP ( 'NONE', ( #2312, #10473, #7213, #131 ) ) ;
#2218=PRODUCT_DEFINITION_SHAPE ( 'NONE', 'NONE',  #6773 ) ;
#2219=EDGE_CURVE ( 'NONE', #288, #9816, #5526, .T. ) ;
#2223=EDGE_LOOP ( 'NONE', ( #3669, #9856, #2555, #8359 ) ) ;
#2230=CARTESIAN_POINT ( 'NONE',  ( -20.29350689640809691, 140.5696653505793563, 20.00000000000002132 ) ) ;
#2235=ADVANCED_FACE ( 'NONE', ( #5810 ), #7567, .F. ) ;
#2238=EDGE_LOOP ( 'NONE', ( #3655, #6176 ) ) ;
#2244=FACE_OUTER_BOUND ( 'NONE', #5322, .T. ) ;
#2245=EDGE_CURVE ( 'NONE', #1079, #7959, #5067, .T. ) ;
#2257=ORIENTED_EDGE ( 'NONE', *, *, #5471, .F. ) ;
#2259=VECTOR ( 'NONE', #9983, 1000.000000000000000 ) ;
#2262=CARTESIAN_POINT ( 'NONE',  ( -7.293506896408097795, 80.56966535057935630, -20.00000000000000711 ) ) ;
#2274=LINE ( 'NONE', #8789, #5355 ) ;
#2290=ORIENTED_EDGE ( 'NONE', *, *, #302, .F. ) ;
#2292=ADVANCED_FACE ( 'NONE', ( #5913 ), #1942, .T. ) ;
#2293=FACE_BOUND ( 'NONE', #2238, .T. ) ;
#2306=EDGE_CURVE ( 'NONE', #4058, #5577, #2145, .T. ) ;
#2312=ORIENTED_EDGE ( 'NONE', *, *, #317, .F. ) ;
#2343=FACE_BOUND ( 'NONE', #1146, .T. ) ;
#2352=VECTOR ( 'NONE', #6005, 1000.000000000000000 ) ;
#2356=CARTESIAN_POINT ( 'NONE',  ( -2.293506896408097795, 37.08684478514406635, 0.000000000000000000 ) ) ;
#2373=LINE ( 'NONE', #9601, #5862 ) ;
#2381=ORIENTED_EDGE ( 'NONE', *, *, #2399, .F. ) ;
#2382=VECTOR ( 'NONE', #6443, 1000.000000000000000 ) ;
#2398=CARTESIAN_POINT ( 'NONE',  ( -7.293506896408097795, 0.000000000000000000, 0.000000000000000000 ) ) ;
#2399=EDGE_CURVE ( 'NONE', #4328, #3441, #1998, .T. ) ;
#2408=AXIS2_PLACEMENT_3D ( 'NONE', #1870, #344, #4153 ) ;
#2409=DIRECTION ( 'NONE',  ( 1.000000000000000000, 0.000000000000000000, 0.000000000000000000 ) ) ;
#2412=ORIENTED_EDGE ( 'NONE', *, *, #2808, .T. ) ;
#2416=FACE_BOUND ( 'NONE', #1291, .T. ) ;
#2419=AXIS2_PLACEMENT_3D ( 'NONE', #9172, #3353, #8112 ) ;
#2420=DIRECTION ( 'NONE',  ( 0.000000000000000000, -1.000000000000000000, 0.000000000000000000 ) ) ;
#2426=LINE ( 'NONE', #8096, #2852 ) ;
#2430=EDGE_CURVE ( 'NONE', #9336, #7089, #4541, .T. ) ;
#2437=ORIENTED_EDGE ( 'NONE', *, *, #4240, .F. ) ;
#2440=DIRECTION ( 'NONE',  ( 1.000000000000000000, -0.000000000000000000, -0.000000000000000000 ) ) ;
#2444=DIRECTION ( 'NONE',  ( -0.000000000000000000, -0.000000000000000000, 1.000000000000000000 ) ) ;
#2445=ORIENTED_EDGE ( 'NONE', *, *, #2306, .F. ) ;
#2446=CARTESIAN_POINT ( 'NONE',  ( -20.29350689640810401, 150.5696653505793563, 10.98204862120179826 ) ) ;
#2447=ORIENTED_EDGE ( 'NONE', *, *, #3925, .F. ) ;
#2451=VERTEX_POINT ( 'NONE', #9474 ) ;
#2457=ORIENTED_EDGE ( 'NONE', *, *, #4077, .F. ) ;
#2464=AXIS2_PLACEMENT_3D ( 'NONE', #935, #8088, #878 ) ;
#2466=FACE_BOUND ( 'NONE', #3000, .T. ) ;
#2469=AXIS2_PLACEMENT_3D ( 'NONE', #4152, #4935, #5894 ) ;
#2475=AXIS2_PLACEMENT_3D ( 'NONE', #6834, #3713, #5342 ) ;
#2479=CARTESIAN_POINT ( 'NONE',  ( -7.293506896408097795, 2.445795361565304815E-15, 20.00000000000002132 ) ) ;
#2483=ORIENTED_EDGE ( 'NONE', *, *, #8314, .F. ) ;
#2484=AXIS2_PLACEMENT_3D ( 'NONE', #3876, #9546, #7106 ) ;
#2485=ORIENTED_EDGE ( 'NONE', *, *, #7022, .F. ) ;
#2487=EDGE_CURVE ( 'NONE', #1403, #5783, #9113, .T. ) ;
#2488=ORIENTED_EDGE ( 'NONE', *, *, #2547, .F. ) ;
#2492=CARTESIAN_POINT ( 'NONE',  ( -30.29350689640809335, 72.56966535057935630, -20.00000000000001066 ) ) ;
#2496=CARTESIAN_POINT ( 'NONE',  ( -16.29350689640809691, -19.43033464942062238, 0.000000000000000000 ) ) ;
#2500=VERTEX_POINT ( 'NONE', #10423 ) ;
#2503=EDGE_CURVE ( 'NONE', #5058, #6356, #3028, .T. ) ;
#2505=ORIENTED_EDGE ( 'NONE', *, *, #5133, .F. ) ;
#2509=DIRECTION ( 'NONE',  ( -0.000000000000000000, 1.000000000000000000, -0.000000000000000000 ) ) ;
#2513=CARTESIAN_POINT ( 'NONE',  ( -30.29350689640809335, 2.445795361565304815E-15, 20.00000000000002132 ) ) ;
#2515=VECTOR ( 'NONE', #35, 1000.000000000000000 ) ;
#2516=CARTESIAN_POINT ( 'NONE',  ( -2.293506896408097795, 80.56966535057935630, -16.00000000000000711 ) ) ;
#2519=ORIENTED_EDGE ( 'NONE', *, *, #7483, .F. ) ;
#2520=CIRCLE ( 'NONE', #4213, 7.999999999999991118 ) ;
#2522=FACE_BOUND ( 'NONE', #7412, .T. ) ;
#2529=DIRECTION ( 'NONE',  ( 0.000000000000000000, -1.000000000000000000, 1.222897680782651224E-16 ) ) ;
#2535=ADVANCED_FACE ( 'NONE', ( #4010 ), #6436, .T. ) ;
#2541=EDGE_LOOP ( 'NONE', ( #2097, #5873, #6376, #4643 ) ) ;
#2543=CARTESIAN_POINT ( 'NONE',  ( -30.29350689640809335, 120.5696653505793705, 24.00000000000000711 ) ) ;
#2547=EDGE_CURVE ( 'NONE', #9480, #6361, #10475, .T. ) ;
#2554=CARTESIAN_POINT ( 'NONE',  ( -20.29350689640810046, 150.5696653505793563, -20.00000000000000355 ) ) ;
#2555=ORIENTED_EDGE ( 'NONE', *, *, #8994, .T. ) ;
#2580=LINE ( 'NONE', #9855, #6127 ) ;
#2581=AXIS2_PLACEMENT_3D ( 'NONE', #3988, #4678, #8705 ) ;
#2590=EDGE_LOOP ( 'NONE', ( #6199, #5120, #6180, #2437, #4980, #9978 ) ) ;
#2598=ORIENTED_EDGE ( 'NONE', *, *, #7222, .F. ) ;
#2607=ORIENTED_EDGE ( 'NONE', *, *, #9637, .F. ) ;
#2613=ORIENTED_EDGE ( 'NONE', *, *, #846, .F. ) ;
#2627=EDGE_CURVE ( 'NONE', #9462, #5715, #6060, .T. ) ;
#2636=DIRECTION ( 'NONE',  ( 0.000000000000000000, 0.000000000000000000, 1.000000000000000000 ) ) ;
#2638=AXIS2_PLACEMENT_3D ( 'NONE', #3741, #7086, #6975 ) ;
#2649=CIRCLE ( 'NONE', #7896, 7.999999999999996447 ) ;
#2658=DIRECTION ( 'NONE',  ( -1.000000000000000000, 0.000000000000000000, 0.000000000000000000 ) ) ;
#2665=CIRCLE ( 'NONE', #7239, 4.000000000000000000 ) ;
#2679=AXIS2_PLACEMENT_3D ( 'NONE', #621, #2409, #3157 ) ;
#2705=CARTESIAN_POINT ( 'NONE',  ( -16.29350689640809691, -19.43033464942062238, -7.500000000000000000 ) ) ;
#2711=DIRECTION ( 'NONE',  ( 1.000000000000000000, 0.000000000000000000, 0.000000000000000000 ) ) ;
#2735=DIRECTION ( 'NONE',  ( 0.000000000000000000, 0.3481865296036273372, 0.9374252720097653313 ) ) ;
#2737=ADVANCED_FACE ( 'NONE', ( #9140 ), #4112, .T. ) ;
#2742=LINE ( 'NONE', #3598, #8452 ) ;
#2743=CARTESIAN_POINT ( 'NONE',  ( -30.29350689640809335, 88.56966535057934209, 20.00000000000001066 ) ) ;
#2764=LINE ( 'NONE', #9236, #5097 ) ;
#2770=ORIENTED_EDGE ( 'NONE', *, *, #7364, .F. ) ;
#2786=ORIENTED_EDGE ( 'NONE', *, *, #10087, .T. ) ;
#2789=ORIENTED_EDGE ( 'NONE', *, *, #5653, .T. ) ;
#2791=DIRECTION ( 'NONE',  ( 0.000000000000000000, -0.9374252720097652203, -0.3481865296036273372 ) ) ;
#2795=DIRECTION ( 'NONE',  ( 0.000000000000000000, 0.000000000000000000, 1.000000000000000000 ) ) ;
#2802=ORIENTED_EDGE ( 'NONE', *, *, #2883, .T. ) ;
#2804=VECTOR ( 'NONE', #4535, 1000.000000000000000 ) ;
#2808=EDGE_CURVE ( 'NONE', #941, #9176, #7767, .T. ) ;
#2810=AXIS2_PLACEMENT_3D ( 'NONE', #2981, #8549, #8601 ) ;
#2812=ORIENTED_EDGE ( 'NONE', *, *, #3269, .T. ) ;
#2813=( LENGTH_UNIT ( ) NAMED_UNIT ( * ) SI_UNIT ( .MILLI., .METRE. ) );
#2816=ORIENTED_EDGE ( 'NONE', *, *, #2872, .T. ) ;
#2818=PLANE ( 'NONE',  #7976 ) ;
#2819=AXIS2_PLACEMENT_3D ( 'NONE', #157, #992, #3382 ) ;
#2823=AXIS2_PLACEMENT_3D ( 'NONE', #5003, #1676, #827 ) ;
#2832=CIRCLE ( 'NONE', #8766, 3.999999999999976019 ) ;
#2844=ORIENTED_EDGE ( 'NONE', *, *, #7010, .F. ) ;
#2845=EDGE_CURVE ( 'NONE', #5058, #6361, #7654, .T. ) ;
#2847=CARTESIAN_POINT ( 'NONE',  ( -30.29350689640809335, 120.5696653505793705, -24.00000000000000711 ) ) ;
#2850=DIRECTION ( 'NONE',  ( 0.000000000000000000, -0.9374252720097652203, 0.3481865296036273372 ) ) ;
#2851=DIRECTION ( 'NONE',  ( 0.000000000000000000, 0.000000000000000000, -1.000000000000000000 ) ) ;
#2852=VECTOR ( 'NONE', #4176, 1000.000000000000000 ) ;
#2854=ORIENTED_EDGE ( 'NONE', *, *, #1220, .F. ) ;
#2855=AXIS2_PLACEMENT_3D ( 'NONE', #4218, #6703, #6546 ) ;
#2868=ORIENTED_EDGE ( 'NONE', *, *, #1888, .T. ) ;
#2872=EDGE_CURVE ( 'NONE', #6085, #6072, #6861, .T. ) ;
#2873=EDGE_CURVE ( 'NONE', #3604, #1439, #7812, .T. ) ;
#2874=CARTESIAN_POINT ( 'NONE',  ( -7.293506896408097795, -3.651280424770854409E-15, 24.99999999999998579 ) ) ;
#2883=EDGE_CURVE ( 'NONE', #6933, #10322, #2520, .T. ) ;
#2885=CARTESIAN_POINT ( 'NONE',  ( -16.29350689640809691, 37.08684478514406635, 0.000000000000000000 ) ) ;
#2897=ORIENTED_EDGE ( 'NONE', *, *, #5173, .T. ) ;
#2899=DIRECTION ( 'NONE',  ( -0.000000000000000000, -0.000000000000000000, 1.000000000000000000 ) ) ;
#2902=CARTESIAN_POINT ( 'NONE',  ( -20.29350689640809691, 140.5696653505793563, 10.98204862120179826 ) ) ;
#2910=CARTESIAN_POINT ( 'NONE',  ( -2.293506896408097795, 80.56966535057935630, 24.00000000000000711 ) ) ;
#2915=AXIS2_PLACEMENT_3D ( 'NONE', #3697, #1302, #10053 ) ;
#2919=EDGE_LOOP ( 'NONE', ( #3689, #3554, #9337, #5592 ) ) ;
#2921=CIRCLE ( 'NONE', #2408, 5.000000000000000888 ) ;
#2923=VERTEX_POINT ( 'NONE', #2554 ) ;
#2927=DIRECTION ( 'NONE',  ( 0.000000000000000000, 0.000000000000000000, 1.000000000000000000 ) ) ;
#2933=EDGE_CURVE ( 'NONE', #6484, #6361, #7434, .T. ) ;
#2937=DIRECTION ( 'NONE',  ( 1.000000000000000000, -0.000000000000000000, -0.000000000000000000 ) ) ;
#2943=EDGE_CURVE ( 'NONE', #3592, #2946, #8102, .T. ) ;
#2946=VERTEX_POINT ( 'NONE', #3358 ) ;
#2948=VERTEX_POINT ( 'NONE', #8918 ) ;
#2952=EDGE_LOOP ( 'NONE', ( #3133, #5885, #5396, #4354, #6897, #7619, #4161, #8812 ) ) ;
#2953=DIRECTION ( 'NONE',  ( 0.000000000000000000, 1.222897680782651471E-16, 1.000000000000000000 ) ) ;
#2962=CARTESIAN_POINT ( 'NONE',  ( -30.29350689640809691, 140.5696653505793563, -10.98204862120179826 ) ) ;
#2981=CARTESIAN_POINT ( 'NONE',  ( -20.29350689640809691, 140.5696653505793563, 20.00000000000002132 ) ) ;
#2984=DIRECTION ( 'NONE',  ( 0.000000000000000000, 0.000000000000000000, -1.000000000000000000 ) ) ;
#2996=PLANE ( 'NONE',  #9928 ) ;
#3000=EDGE_LOOP ( 'NONE', ( #10312, #7315 ) ) ;
#3004=ORIENTED_EDGE ( 'NONE', *, *, #2121, .F. ) ;
#3013=CIRCLE ( 'NONE', #8931, 4.000000000000000000 ) ;
#3025=CARTESIAN_POINT ( 'NONE',  ( -7.293506896408097795, 72.08684478514406635, 28.00000000000001066 ) ) ;
#3027=CYLINDRICAL_SURFACE ( 'NONE', #6512, 3.999999999999989786 ) ;
#3028=CIRCLE ( 'NONE', #4380, 7.999999999999994671 ) ;
#3037=CARTESIAN_POINT ( 'NONE',  ( -2.293506896408097795, 145.5696653505793563, -20.00000000000000711 ) ) ;
#3047=DIRECTION ( 'NONE',  ( 1.000000000000000000, -0.000000000000000000, -0.000000000000000000 ) ) ;
#3052=ORIENTED_EDGE ( 'NONE', *, *, #8775, .T. ) ;
#3056=PLANE ( 'NONE',  #9068 ) ;
#3058=DIRECTION ( 'NONE',  ( 0.000000000000000000, 0.000000000000000000, -1.000000000000000000 ) ) ;
#3061=CARTESIAN_POINT ( 'NONE',  ( -30.29350689640809335, 0.000000000000000000, -10.98204862120179826 ) ) ;
#3077=MANIFOLD_SOLID_BREP ( 'Move Face4', #9619 ) ;
#3083=VERTEX_POINT ( 'NONE', #7485 ) ;
#3091=CARTESIAN_POINT ( 'NONE',  ( -2.293506896408097795, 72.08684478514408056, -28.00000000000001421 ) ) ;
#3097=DIRECTION ( 'NONE',  ( 0.000000000000000000, 0.000000000000000000, -1.000000000000000000 ) ) ;
#3105=DIRECTION ( 'NONE',  ( 0.000000000000000000, 0.000000000000000000, 1.000000000000000000 ) ) ;
#3107=EDGE_LOOP ( 'NONE', ( #3650, #6315, #5449, #2149 ) ) ;
#3114=DIRECTION ( 'NONE',  ( -1.000000000000000000, 0.000000000000000000, 0.000000000000000000 ) ) ;
#3124=LINE ( 'NONE', #6357, #7841 ) ;
#3133=ORIENTED_EDGE ( 'NONE', *, *, #3738, .F. ) ;
#3142=ORIENTED_EDGE ( 'NONE', *, *, #3738, .T. ) ;
#3145=ORIENTED_EDGE ( 'NONE', *, *, #9615, .F. ) ;
#3146=EDGE_CURVE ( 'NONE', #1352, #6365, #8791, .T. ) ;
#3148=VECTOR ( 'NONE', #8062, 1000.000000000000000 ) ;
#3151=LINE ( 'NONE', #2356, #2804 ) ;
#3157=DIRECTION ( 'NONE',  ( 0.000000000000000000, 0.000000000000000000, -1.000000000000000000 ) ) ;
#3168=ORIENTED_EDGE ( 'NONE', *, *, #2125, .T. ) ;
#3172=EDGE_LOOP ( 'NONE', ( #7911, #8752, #2488, #3981 ) ) ;
#3175=ORIENTED_EDGE ( 'NONE', *, *, #6434, .F. ) ;
#3181=ORIENTED_EDGE ( 'NONE', *, *, #6146, .T. ) ;
#3187=ORIENTED_EDGE ( 'NONE', *, *, #2933, .F. ) ;
#3190=CIRCLE ( 'NONE', #1837, 7.999999999999991118 ) ;
#3194=EDGE_CURVE ( 'NONE', #5730, #5162, #945, .T. ) ;
#3202=FACE_OUTER_BOUND ( 'NONE', #6399, .T. ) ;
#3214=DIRECTION ( 'NONE',  ( 1.000000000000000000, 0.000000000000000000, 0.000000000000000000 ) ) ;
#3225=EDGE_CURVE ( 'NONE', #3083, #1282, #10064, .T. ) ;
#3235=VECTOR ( 'NONE', #3947, 1000.000000000000000 ) ;
#3237=CYLINDRICAL_SURFACE ( 'NONE', #2581, 4.000000000000000000 ) ;
#3239=CARTESIAN_POINT ( 'NONE',  ( -7.293506896408098683, 126.8146633489777599, -25.00000000000000355 ) ) ;
#3255=SHAPE_DEFINITION_REPRESENTATION ( #2218, #6561 ) ;
#3269=EDGE_CURVE ( 'NONE', #3083, #9462, #2742, .T. ) ;
#3270=DIRECTION ( 'NONE',  ( 0.000000000000000000, 1.000000000000000000, 1.460512169908342690E-16 ) ) ;
#3277=CARTESIAN_POINT ( 'NONE',  ( -30.29350689640809335, 120.5696653505793705, -20.00000000000000711 ) ) ;
#3278=VECTOR ( 'NONE', #10445, 1000.000000000000000 ) ;
#3288=EDGE_LOOP ( 'NONE', ( #4401, #5969, #4608, #8237 ) ) ;
#3289=LINE ( 'NONE', #2492, #316 ) ;
#3316=EDGE_LOOP ( 'NONE', ( #339, #4105, #5227, #8693 ) ) ;
#3317=DIRECTION ( 'NONE',  ( 0.000000000000000000, -1.000000000000000000, -1.222897680782651471E-16 ) ) ;
#3320=DIRECTION ( 'NONE',  ( 0.000000000000000000, 0.000000000000000000, 1.000000000000000000 ) ) ;
#3327=DIRECTION ( 'NONE',  ( 0.000000000000000000, -0.9374252720097653313, -0.3481865296036273372 ) ) ;
#3334=CARTESIAN_POINT ( 'NONE',  ( -2.293506896408097795, 120.5696653505793705, -20.00000000000000711 ) ) ;
#3335=AXIS2_PLACEMENT_3D ( 'NONE', #3451, #2658, #9880 ) ;
#3343=ORIENTED_EDGE ( 'NONE', *, *, #856, .F. ) ;
#3347=ORIENTED_EDGE ( 'NONE', *, *, #1454, .T. ) ;
#3352=APPLICATION_CONTEXT ( 'automotive_design' ) ;
#3353=DIRECTION ( 'NONE',  ( -1.000000000000000000, 0.000000000000000000, 0.000000000000000000 ) ) ;
#3357=ORIENTED_EDGE ( 'NONE', *, *, #4109, .F. ) ;
#3358=CARTESIAN_POINT ( 'NONE',  ( -30.29350689640809335, 80.56966535057935630, 16.00000000000000711 ) ) ;
#3363=PLANE ( 'NONE',  #2469 ) ;
#3378=PLANE ( 'NONE',  #6960 ) ;
#3382=DIRECTION ( 'NONE',  ( 0.000000000000000000, 0.000000000000000000, 1.000000000000000000 ) ) ;
#3384=CARTESIAN_POINT ( 'NONE',  ( -2.293506896408097795, 120.5696653505793705, -20.00000000000000711 ) ) ;
#3391=ORIENTED_EDGE ( 'NONE', *, *, #2219, .T. ) ;
#3396=CARTESIAN_POINT ( 'NONE',  ( -30.29350689640809335, 120.5696653505793705, 20.00000000000000711 ) ) ;
#3397=DIRECTION ( 'NONE',  ( -1.000000000000000000, 0.000000000000000000, 0.000000000000000000 ) ) ;
#3403=VERTEX_POINT ( 'NONE', #10332 ) ;
#3407=ORIENTED_EDGE ( 'NONE', *, *, #6053, .T. ) ;
#3410=CARTESIAN_POINT ( 'NONE',  ( -2.293506896408097795, 0.000000000000000000, 10.98204862120179826 ) ) ;
#3411=DIRECTION ( 'NONE',  ( -0.000000000000000000, -0.000000000000000000, 1.000000000000000000 ) ) ;
#3414=ADVANCED_FACE ( 'NONE', ( #9591 ), #5389, .T. ) ;
#3441=VERTEX_POINT ( 'NONE', #3753 ) ;
#3446=DIRECTION ( 'NONE',  ( 0.000000000000000000, -1.000000000000000000, 1.431206729101514631E-16 ) ) ;
#3448=CYLINDRICAL_SURFACE ( 'NONE', #4857, 7.500000000000000000 ) ;
#3451=CARTESIAN_POINT ( 'NONE',  ( -7.293506896408097795, 0.000000000000000000, 0.000000000000000000 ) ) ;
#3474=ADVANCED_FACE ( 'NONE', ( #5803, #2466, #9688, #2416, #5645 ), #4898, .T. ) ;
#3475=AXIS2_PLACEMENT_3D ( 'NONE', #7943, #9593, #5391 ) ;
#3488=AXIS2_PLACEMENT_3D ( 'NONE', #5331, #6237, #4544 ) ;
#3491=CARTESIAN_POINT ( 'NONE',  ( -30.29350689640809335, 88.56966535057934209, -20.00000000000001066 ) ) ;
#3494=EDGE_CURVE ( 'NONE', #6362, #10164, #5867, .T. ) ;
#3514=DIRECTION ( 'NONE',  ( -0.000000000000000000, -0.000000000000000000, 1.000000000000000000 ) ) ;
#3518=DIRECTION ( 'NONE',  ( 0.000000000000000000, 1.000000000000000000, -0.000000000000000000 ) ) ;
#3519=FACE_OUTER_BOUND ( 'NONE', #5635, .T. ) ;
#3523=ADVANCED_FACE ( 'NONE', ( #2522, #5748 ), #4115, .F. ) ;
#3527=ADVANCED_FACE ( 'NONE', ( #9905 ), #8031, .F. ) ;
#3547=LINE ( 'NONE', #418, #9530 ) ;
#3550=FACE_OUTER_BOUND ( 'NONE', #5042, .T. ) ;
#3551=CARTESIAN_POINT ( 'NONE',  ( -30.29350689640809335, 50.54838324668256888, -20.00000000000001776 ) ) ;
#3554=ORIENTED_EDGE ( 'NONE', *, *, #8653, .T. ) ;
#3560=LINE ( 'NONE', #10028, #10302 ) ;
#3562=DIRECTION ( 'NONE',  ( 0.000000000000000000, 0.000000000000000000, 1.000000000000000000 ) ) ;
#3571=ORIENTED_EDGE ( 'NONE', *, *, #1516, .T. ) ;
#3592=VERTEX_POINT ( 'NONE', #7504 ) ;
#3596=ADVANCED_FACE ( 'NONE', ( #6707 ), #6864, .T. ) ;
#3598=CARTESIAN_POINT ( 'NONE',  ( 67.68113203623319407, 150.5696653505793563, -10.98204862120179826 ) ) ;
#3600=DIRECTION ( 'NONE',  ( -0.000000000000000000, -0.000000000000000000, 1.000000000000000000 ) ) ;
#3604=VERTEX_POINT ( 'NONE', #6808 ) ;
#3631=CARTESIAN_POINT ( 'NONE',  ( -20.29350689640809691, 140.5696653505793563, 19.97500000000000853 ) ) ;
#3637=PLANE ( 'NONE',  #7469 ) ;
#3638=ORIENTED_EDGE ( 'NONE', *, *, #5713, .T. ) ;
#3643=ORIENTED_EDGE ( 'NONE', *, *, #3269, .F. ) ;
#3650=ORIENTED_EDGE ( 'NONE', *, *, #9181, .F. ) ;
#3652=FACE_BOUND ( 'NONE', #3826, .T. ) ;
#3655=ORIENTED_EDGE ( 'NONE', *, *, #2306, .T. ) ;
#3669=ORIENTED_EDGE ( 'NONE', *, *, #1353, .F. ) ;
#3673=EDGE_CURVE ( 'NONE', #6943, #1359, #7133, .T. ) ;
#3689=ORIENTED_EDGE ( 'NONE', *, *, #2430, .F. ) ;
#3697=CARTESIAN_POINT ( 'NONE',  ( -30.29350689640809335, 80.56966535057935630, -20.00000000000000711 ) ) ;
#3702=ORIENTED_EDGE ( 'NONE', *, *, #7765, .T. ) ;
#3708=CIRCLE ( 'NONE', #7424, 4.000000000000000000 ) ;
#3713=DIRECTION ( 'NONE',  ( 1.000000000000000000, -0.000000000000000000, -0.000000000000000000 ) ) ;
#3720=CARTESIAN_POINT ( 'NONE',  ( -7.293506896408097795, 126.8146633489777599, -25.00000000000000355 ) ) ;
#3734=DIRECTION ( 'NONE',  ( 1.000000000000000000, -0.000000000000000000, -0.000000000000000000 ) ) ;
#3735=EDGE_LOOP ( 'NONE', ( #6413, #7623, #2173, #5422, #9244 ) ) ;
#3738=EDGE_CURVE ( 'NONE', #1083, #9488, #10156, .T. ) ;
#3739=LINE ( 'NONE', #6972, #7917 ) ;
#3741=CARTESIAN_POINT ( 'NONE',  ( -7.293506896408097795, 120.5696653505793705, 20.00000000000000711 ) ) ;
#3743=CARTESIAN_POINT ( 'NONE',  ( -7.293506896408097795, 120.5696653505793705, -28.00000000000000355 ) ) ;
#3750=FACE_OUTER_BOUND ( 'NONE', #4998, .T. ) ;
#3753=CARTESIAN_POINT ( 'NONE',  ( -7.293506896408097795, 88.56966535057934209, -20.00000000000001066 ) ) ;
#3758=CIRCLE ( 'NONE', #1552, 4.000000000000000000 ) ;
#3760=EDGE_CURVE ( 'NONE', #1079, #4081, #9522, .T. ) ;
#3762=ORIENTED_EDGE ( 'NONE', *, *, #6804, .T. ) ;
#3770=CARTESIAN_POINT ( 'NONE',  ( -30.29350689640809335, 140.5696653505793563, 10.98204862120180003 ) ) ;
#3771=LINE ( 'NONE', #9080, #9739 ) ;
#3782=CARTESIAN_POINT ( 'NONE',  ( -7.293506896408097795, 2.445795361565304815E-15, 20.00000000000002132 ) ) ;
#3787=EDGE_CURVE ( 'NONE', #941, #4587, #3739, .T. ) ;
#3796=CIRCLE ( 'NONE', #6342, 7.500000000000000000 ) ;
#3805=AXIS2_PLACEMENT_3D ( 'NONE', #4210, #3411, #7282 ) ;
#3814=CARTESIAN_POINT ( 'NONE',  ( -30.29350689640809335, 88.56966535057934209, 20.00000000000001066 ) ) ;
#3822=DIRECTION ( 'NONE',  ( 0.000000000000000000, 0.000000000000000000, 1.000000000000000000 ) ) ;
#3823=EDGE_CURVE ( 'NONE', #6283, #1352, #5884, .T. ) ;
#3824=DIRECTION ( 'NONE',  ( 0.000000000000000000, -1.000000000000000000, 1.431206729101514631E-16 ) ) ;
#3826=EDGE_LOOP ( 'NONE', ( #3391, #3168 ) ) ;
#3830=EDGE_LOOP ( 'NONE', ( #5465, #4515, #7641, #5821 ) ) ;
#3832=PLANE ( 'NONE',  #5211 ) ;
#3841=CARTESIAN_POINT ( 'NONE',  ( -7.293506896408097795, 4.007378841484243628E-15, -28.00000000000002132 ) ) ;
#3845=VECTOR ( 'NONE', #10030, 1000.000000000000000 ) ;
#3846=AXIS2_PLACEMENT_3D ( 'NONE', #8134, #1728, #8881 ) ;
#3852=ADVANCED_FACE ( 'NONE', ( #279 ), #1861, .F. ) ;
#3862=CARTESIAN_POINT ( 'NONE',  ( -30.29350689640809335, 72.56966535057935630, 20.00000000000001066 ) ) ;
#3870=ADVANCED_FACE ( 'NONE', ( #5773 ), #3448, .F. ) ;
#3873=AXIS2_PLACEMENT_3D ( 'NONE', #9544, #4707, #2636 ) ;
#3874=AXIS2_PLACEMENT_3D ( 'NONE', #4933, #3514, #2711 ) ;
#3876=CARTESIAN_POINT ( 'NONE',  ( -20.29350689640809691, 140.5696653505793563, -10.98204862120179648 ) ) ;
#3895=DIRECTION ( 'NONE',  ( 1.000000000000000000, -0.000000000000000000, -0.000000000000000000 ) ) ;
#3896=LINE ( 'NONE', #7965, #4171 ) ;
#3900=EDGE_CURVE ( 'NONE', #9176, #5189, #1116, .T. ) ;
#3902=CARTESIAN_POINT ( 'NONE',  ( -16.29350689640809691, 55.56966535057936341, 7.500000000000000000 ) ) ;
#3912=ORIENTED_EDGE ( 'NONE', *, *, #1220, .T. ) ;
#3918=DIRECTION ( 'NONE',  ( 0.000000000000000000, 1.000000000000000000, -0.000000000000000000 ) ) ;
#3919=CARTESIAN_POINT ( 'NONE',  ( -7.293506896408097795, 72.56966535057935630, 20.00000000000001066 ) ) ;
#3925=EDGE_CURVE ( 'NONE', #2500, #4525, #2665, .T. ) ;
#3941=DIRECTION ( 'NONE',  ( 0.000000000000000000, -1.000000000000000000, 1.431206729101514631E-16 ) ) ;
#3947=DIRECTION ( 'NONE',  ( 0.000000000000000000, -1.000000000000000000, -1.431206729101514631E-16 ) ) ;
#3959=EDGE_LOOP ( 'NONE', ( #1776, #272, #2483, #1311, #1653 ) ) ;
#3967=CARTESIAN_POINT ( 'NONE',  ( -20.29350689640809691, 140.5696653505793563, 20.00000000000002132 ) ) ;
#3972=ORIENTED_EDGE ( 'NONE', *, *, #8828, .T. ) ;
#3973=CARTESIAN_POINT ( 'NONE',  ( -16.29350689640810401, 140.5696653505793563, 19.97500000000000853 ) ) ;
#3975=CARTESIAN_POINT ( 'NONE',  ( -30.29350689640809335, 50.54838324668256888, 20.00000000000001776 ) ) ;
#3981=ORIENTED_EDGE ( 'NONE', *, *, #1380, .F. ) ;
#3985=FACE_OUTER_BOUND ( 'NONE', #4682, .T. ) ;
#3988=CARTESIAN_POINT ( 'NONE',  ( -30.29350689640809335, 120.5696653505793705, -20.00000000000000711 ) ) ;
#4001=AXIS2_PLACEMENT_3D ( 'NONE', #7758, #3734, #2984 ) ;
#4007=CIRCLE ( 'NONE', #2475, 7.999999999999991118 ) ;
#4010=FACE_OUTER_BOUND ( 'NONE', #7372, .T. ) ;
#4018=LINE ( 'NONE', #7188, #2382 ) ;
#4020=FACE_OUTER_BOUND ( 'NONE', #97, .T. ) ;
#4025=VERTEX_POINT ( 'NONE', #1225 ) ;
#4031=ORIENTED_EDGE ( 'NONE', *, *, #10339, .F. ) ;
#4040=DIRECTION ( 'NONE',  ( 0.000000000000000000, 0.000000000000000000, 1.000000000000000000 ) ) ;
#4042=CARTESIAN_POINT ( 'NONE',  ( -30.29350689640809335, 80.56966535057935630, -16.00000000000000711 ) ) ;
#4056=ORIENTED_EDGE ( 'NONE', *, *, #2503, .T. ) ;
#4058=VERTEX_POINT ( 'NONE', #6842 ) ;
#4071=DIRECTION ( 'NONE',  ( 0.000000000000000000, 0.000000000000000000, 1.000000000000000000 ) ) ;
#4077=EDGE_CURVE ( 'NONE', #716, #1117, #3013, .T. ) ;
#4081=VERTEX_POINT ( 'NONE', #3770 ) ;
#4088=CARTESIAN_POINT ( 'NONE',  ( -2.293506896408097795, -3.651280424770854409E-15, -24.99999999999998579 ) ) ;
#4093=EDGE_CURVE ( 'NONE', #596, #8054, #3560, .T. ) ;
#4098=DIRECTION ( 'NONE',  ( -0.000000000000000000, -0.000000000000000000, 1.000000000000000000 ) ) ;
#4105=ORIENTED_EDGE ( 'NONE', *, *, #4077, .T. ) ;
#4108=EDGE_CURVE ( 'NONE', #5466, #6943, #7744, .T. ) ;
#4109=EDGE_CURVE ( 'NONE', #2019, #3592, #3, .T. ) ;
#4110=ORIENTED_EDGE ( 'NONE', *, *, #8133, .F. ) ;
#4112=CYLINDRICAL_SURFACE ( 'NONE', #2855, 7.999999999999996447 ) ;
#4114=ORIENTED_EDGE ( 'NONE', *, *, #1786, .F. ) ;
#4115=PLANE ( 'NONE',  #8924 ) ;
#4124=DIRECTION ( 'NONE',  ( -0.000000000000000000, -0.000000000000000000, -1.000000000000000000 ) ) ;
#4138=CARTESIAN_POINT ( 'NONE',  ( -2.293506896408097795, 80.56966535057935630, 20.00000000000000711 ) ) ;
#4150=CARTESIAN_POINT ( 'NONE',  ( -7.293506896408097795, -3.651280424770854409E-15, -24.99999999999998579 ) ) ;
#4152=CARTESIAN_POINT ( 'NONE',  ( -30.29350689640809335, 2.445795361565304815E-15, -20.00000000000002132 ) ) ;
#4153=DIRECTION ( 'NONE',  ( 0.000000000000000000, 0.000000000000000000, 1.000000000000000000 ) ) ;
#4161=ORIENTED_EDGE ( 'NONE', *, *, #5909, .T. ) ;
#4164=ADVANCED_FACE ( 'NONE', ( #7955 ), #7903, .T. ) ;
#4165=DIRECTION ( 'NONE',  ( -0.000000000000000000, 1.000000000000000000, -0.000000000000000000 ) ) ;
#4171=VECTOR ( 'NONE', #8652, 1000.000000000000000 ) ;
#4176=DIRECTION ( 'NONE',  ( -0.000000000000000000, -0.000000000000000000, 1.000000000000000000 ) ) ;
#4188=EDGE_LOOP ( 'NONE', ( #7960, #1571, #4512, #5298 ) ) ;
#4195=DIRECTION ( 'NONE',  ( 0.000000000000000000, -1.000000000000000000, 1.222897680782651224E-16 ) ) ;
#4198=DIRECTION ( 'NONE',  ( 1.000000000000000000, -0.000000000000000000, -0.000000000000000000 ) ) ;
#4210=CARTESIAN_POINT ( 'NONE',  ( -20.29350689640809691, 140.5696653505793563, 20.00000000000002132 ) ) ;
#4213=AXIS2_PLACEMENT_3D ( 'NONE', #5315, #1983, #1190 ) ;
#4218=CARTESIAN_POINT ( 'NONE',  ( -30.29350689640809335, 80.56966535057935630, -20.00000000000000711 ) ) ;
#4220=MECHANICAL_DESIGN_GEOMETRIC_PRESENTATION_REPRESENTATION('',(#9306),#1003);
#4229=DIRECTION ( 'NONE',  ( 0.000000000000000000, -0.9374252720097653313, 0.3481865296036273372 ) ) ;
#4240=EDGE_CURVE ( 'NONE', #7054, #5162, #1541, .T. ) ;
#4242=FACE_OUTER_BOUND ( 'NONE', #3735, .T. ) ;
#4244=DIRECTION ( 'NONE',  ( -0.000000000000000000, 1.000000000000000000, -0.000000000000000000 ) ) ;
#4246=ORIENTED_EDGE ( 'NONE', *, *, #4093, .T. ) ;
#4261=VERTEX_POINT ( 'NONE', #4910 ) ;
#4282=LINE ( 'NONE', #1157, #1897 ) ;
#4284=CARTESIAN_POINT ( 'NONE',  ( -2.293506896408097795, 145.5696653505793563, -25.00000000000000711 ) ) ;
#4292=CARTESIAN_POINT ( 'NONE',  ( -30.29350689640809335, 128.5696653505793563, -20.00000000000000711 ) ) ;
#4317=AXIS2_PLACEMENT_3D ( 'NONE', #1105, #5338, #7782 ) ;
#4321=( NAMED_UNIT ( * ) SI_UNIT ( $, .STERADIAN. ) SOLID_ANGLE_UNIT ( ) );
#4322=CONICAL_SURFACE ( 'NONE', #4665, 4.025000000000000355, 0.7853981633973787790 ) ;
#4327=CARTESIAN_POINT ( 'NONE',  ( -7.293506896408097795, 0.000000000000000000, 0.000000000000000000 ) ) ;
#4328=VERTEX_POINT ( 'NONE', #3491 ) ;
#4329=DIRECTION ( 'NONE',  ( 1.000000000000000000, -0.000000000000000000, -0.000000000000000000 ) ) ;
#4335=ORIENTED_EDGE ( 'NONE', *, *, #7994, .T. ) ;
#4338=CIRCLE ( 'NONE', #7377, 3.999999999999993339 ) ;
#4340=CYLINDRICAL_SURFACE ( 'NONE', #4317, 10.00000000000000000 ) ;
#4344=ORIENTED_EDGE ( 'NONE', *, *, #2245, .T. ) ;
#4354=ORIENTED_EDGE ( 'NONE', *, *, #1888, .F. ) ;
#4361=VERTEX_POINT ( 'NONE', #9003 ) ;
#4362=DIRECTION ( 'NONE',  ( 0.000000000000000000, 1.222897680782651471E-16, 1.000000000000000000 ) ) ;
#4380=AXIS2_PLACEMENT_3D ( 'NONE', #2262, #8670, #3105 ) ;
#4385=DIRECTION ( 'NONE',  ( 0.000000000000000000, 1.222897680782651471E-16, 1.000000000000000000 ) ) ;
#4394=CARTESIAN_POINT ( 'NONE',  ( -7.293506896408097795, -0.3998014571812398832, 1.076388538564875708 ) ) ;
#4396=CARTESIAN_POINT ( 'NONE',  ( -2.293506896408097795, 80.56966535057935630, -20.00000000000000711 ) ) ;
#4401=ORIENTED_EDGE ( 'NONE', *, *, #6630, .T. ) ;
#4402=ORIENTED_EDGE ( 'NONE', *, *, #993, .F. ) ;
#4424=CARTESIAN_POINT ( 'NONE',  ( -30.29350689640809335, 80.56966535057935630, 20.00000000000000711 ) ) ;
#4426=FACE_OUTER_BOUND ( 'NONE', #4188, .T. ) ;
#4428=ADVANCED_FACE ( 'NONE', ( #3550 ), #4340, .T. ) ;
#4449=CIRCLE ( 'NONE', #2915, 7.999999999999994671 ) ;
#4453=CIRCLE ( 'NONE', #8679, 4.000000000000000000 ) ;
#4455=CARTESIAN_POINT ( 'NONE',  ( -30.29350689640809335, 112.5696653505793705, 20.00000000000000711 ) ) ;
#4456=CARTESIAN_POINT ( 'NONE',  ( -7.293506896408097795, 150.5696653505793563, -20.00000000000000711 ) ) ;
#4457=CARTESIAN_POINT ( 'NONE',  ( -30.29350689640809335, 128.5696653505793847, 20.00000000000000711 ) ) ;
#4463=EDGE_CURVE ( 'NONE', #8767, #2192, #10063, .T. ) ;
#4467=DIRECTION ( 'NONE',  ( 0.000000000000000000, -1.000000000000000000, -1.431206729101514631E-16 ) ) ;
#4468=VECTOR ( 'NONE', #2850, 1000.000000000000114 ) ;
#4471=PRODUCT_DEFINITION_FORMATION_WITH_SPECIFIED_SOURCE ( 'ANY', '', #8815, .NOT_KNOWN. ) ;
#4478=CIRCLE ( 'NONE', #750, 10.00000000000000000 ) ;
#4488=ADVANCED_FACE ( 'NONE', ( #3652, #9217 ), #1265, .F. ) ;
#4489=ORIENTED_EDGE ( 'NONE', *, *, #1683, .F. ) ;
#4491=DIRECTION ( 'NONE',  ( 1.000000000000000000, -0.000000000000000000, -0.000000000000000000 ) ) ;
#4501=EDGE_CURVE ( 'NONE', #13, #2946, #6829, .T. ) ;
#4502=ADVANCED_FACE ( 'NONE', ( #1318 ), #7575, .F. ) ;
#4505=ORIENTED_EDGE ( 'NONE', *, *, #7658, .F. ) ;
#4512=ORIENTED_EDGE ( 'NONE', *, *, #4109, .T. ) ;
#4515=ORIENTED_EDGE ( 'NONE', *, *, #9181, .T. ) ;
#4521=LINE ( 'NONE', #2874, #6544 ) ;
#4525=VERTEX_POINT ( 'NONE', #9324 ) ;
#4534=ADVANCED_FACE ( 'NONE', ( #1160 ), #4322, .F. ) ;
#4535=DIRECTION ( 'NONE',  ( 0.000000000000000000, 0.000000000000000000, -1.000000000000000000 ) ) ;
#4540=AXIS2_PLACEMENT_3D ( 'NONE', #8476, #1111, #5137 ) ;
#4541=LINE ( 'NONE', #9419, #121 ) ;
#4544=DIRECTION ( 'NONE',  ( 0.000000000000000000, 0.000000000000000000, 1.000000000000000000 ) ) ;
#4547=DIRECTION ( 'NONE',  ( 0.000000000000000000, 0.000000000000000000, 1.000000000000000000 ) ) ;
#4548=CARTESIAN_POINT ( 'NONE',  ( -30.29350689640809335, 150.5696653505793563, 0.000000000000000000 ) ) ;
#4560=PLANE ( 'NONE',  #1597 ) ;
#4564=ADVANCED_FACE ( 'NONE', ( #7248 ), #5598, .F. ) ;
#4578=DIRECTION ( 'NONE',  ( 0.000000000000000000, -0.9374252720097652203, -0.3481865296036273372 ) ) ;
#4583=VECTOR ( 'NONE', #2420, 1000.000000000000000 ) ;
#4587=VERTEX_POINT ( 'NONE', #1370 ) ;
#4601=AXIS2_PLACEMENT_3D ( 'NONE', #8586, #5983, #5928 ) ;
#4602=ORIENTED_EDGE ( 'NONE', *, *, #4108, .T. ) ;
#4604=ORIENTED_EDGE ( 'NONE', *, *, #1199, .T. ) ;
#4608=ORIENTED_EDGE ( 'NONE', *, *, #1594, .F. ) ;
#4617=VERTEX_POINT ( 'NONE', #6347 ) ;
#4623=CARTESIAN_POINT ( 'NONE',  ( -2.293506896408097795, 80.56966535057935630, 20.00000000000000711 ) ) ;
#4624=CIRCLE ( 'NONE', #61, 4.000000000000000000 ) ;
#4643=ORIENTED_EDGE ( 'NONE', *, *, #303, .T. ) ;
#4665=AXIS2_PLACEMENT_3D ( 'NONE', #372, #3600, #5284 ) ;
#4670=VECTOR ( 'NONE', #9838, 1000.000000000000000 ) ;
#4676=CARTESIAN_POINT ( 'NONE',  ( 0.000000000000000000, 55.56966535057937051, 0.000000000000000000 ) ) ;
#4678=DIRECTION ( 'NONE',  ( 1.000000000000000000, -0.000000000000000000, -0.000000000000000000 ) ) ;
#4682=EDGE_LOOP ( 'NONE', ( #3571, #5451, #72, #438 ) ) ;
#4686=EDGE_LOOP ( 'NONE', ( #6123, #4604, #4489, #3142 ) ) ;
#4688=VECTOR ( 'NONE', #7026, 1000.000000000000000 ) ;
#4696=EDGE_CURVE ( 'NONE', #1043, #195, #9922, .T. ) ;
#4702=CARTESIAN_POINT ( 'NONE',  ( -2.293506896408097795, 55.56966535057937051, 0.000000000000000000 ) ) ;
#4704=DIRECTION ( 'NONE',  ( 0.000000000000000000, 0.000000000000000000, 1.000000000000000000 ) ) ;
#4707=DIRECTION ( 'NONE',  ( 1.000000000000000000, -0.000000000000000000, -0.000000000000000000 ) ) ;
#4708=CIRCLE ( 'NONE', #5373, 4.000000000000000000 ) ;
#4712=FACE_OUTER_BOUND ( 'NONE', #2919, .T. ) ;
#4716=DIRECTION ( 'NONE',  ( -1.000000000000000000, 0.000000000000000000, 0.000000000000000000 ) ) ;
#4726=FACE_OUTER_BOUND ( 'NONE', #675, .T. ) ;
#4736=ORIENTED_EDGE ( 'NONE', *, *, #2873, .T. ) ;
#4740=EDGE_LOOP ( 'NONE', ( #1593, #2485, #2897, #5436 ) ) ;
#4757=ADVANCED_FACE ( 'NONE', ( #1036 ), #8940, .F. ) ;
#4761=AXIS2_PLACEMENT_3D ( 'NONE', #10344, #4716, #737 ) ;
#4771=EDGE_CURVE ( 'NONE', #2451, #10264, #9242, .T. ) ;
#4783=VECTOR ( 'NONE', #4195, 1000.000000000000000 ) ;
#4788=VECTOR ( 'NONE', #8951, 1000.000000000000000 ) ;
#4790=EDGE_LOOP ( 'NONE', ( #8529, #8085, #7990, #3638 ) ) ;
#4792=ORIENTED_EDGE ( 'NONE', *, *, #7994, .F. ) ;
#4799=CARTESIAN_POINT ( 'NONE',  ( -30.29350689640809335, 0.000000000000000000, 10.98204862120179826 ) ) ;
#4819=FACE_BOUND ( 'NONE', #8837, .T. ) ;
#4820=DIRECTION ( 'NONE',  ( 0.000000000000000000, -0.000000000000000000, 1.000000000000000000 ) ) ;
#4830=ORIENTED_EDGE ( 'NONE', *, *, #7222, .T. ) ;
#4831=ORIENTED_EDGE ( 'NONE', *, *, #9472, .F. ) ;
#4837=CARTESIAN_POINT ( 'NONE',  ( -2.293506896408097795, 150.5696653505793563, -20.00000000000000711 ) ) ;
#4844=ORIENTED_EDGE ( 'NONE', *, *, #3760, .F. ) ;
#4850=CARTESIAN_POINT ( 'NONE',  ( -16.29350689640809691, 55.56966535057936341, 0.000000000000000000 ) ) ;
#4852=VECTOR ( 'NONE', #2937, 1000.000000000000000 ) ;
#4854=ORIENTED_EDGE ( 'NONE', *, *, #7278, .T. ) ;
#4857=AXIS2_PLACEMENT_3D ( 'NONE', #2496, #4244, #8324 ) ;
#4859=CARTESIAN_POINT ( 'NONE',  ( -7.293506896408097795, 145.5696653505793563, 25.00000000000000711 ) ) ;
#4876=ADVANCED_FACE ( 'NONE', ( #4426 ), #355, .F. ) ;
#4880=LINE ( 'NONE', #4042, #10109 ) ;
#4898=PLANE ( 'NONE',  #2823 ) ;
#4910=CARTESIAN_POINT ( 'NONE',  ( -7.293506896408098683, 120.5696653505793705, 28.00000000000000355 ) ) ;
#4922=CARTESIAN_POINT ( 'NONE',  ( -2.293506896408097795, 120.5696653505793705, -20.00000000000000711 ) ) ;
#4923=ORIENTED_EDGE ( 'NONE', *, *, #5784, .F. ) ;
#4933=CARTESIAN_POINT ( 'NONE',  ( -20.29350689640809691, 140.5696653505793563, 20.00000000000002132 ) ) ;
#4934=LINE ( 'NONE', #6535, #1719 ) ;
#4935=DIRECTION ( 'NONE',  ( 0.000000000000000000, -1.222897680782651471E-16, 1.000000000000000000 ) ) ;
#4938=VECTOR ( 'NONE', #4329, 1000.000000000000000 ) ;
#4954=CARTESIAN_POINT ( 'NONE',  ( -24.29350689640808625, 140.5696653505793563, -10.98204862120179648 ) ) ;
#4956=ORIENTED_EDGE ( 'NONE', *, *, #7719, .F. ) ;
#4957=EDGE_CURVE ( 'NONE', #39, #4985, #3151, .T. ) ;
#4977=EDGE_CURVE ( 'NONE', #822, #510, #6382, .T. ) ;
#4980=ORIENTED_EDGE ( 'NONE', *, *, #17, .T. ) ;
#4981=LINE ( 'NONE', #6525, #295 ) ;
#4985=VERTEX_POINT ( 'NONE', #10368 ) ;
#4998=EDGE_LOOP ( 'NONE', ( #8517, #5606, #8562, #4110 ) ) ;
#5003=CARTESIAN_POINT ( 'NONE',  ( -30.29350689640809335, 0.000000000000000000, 0.000000000000000000 ) ) ;
#5006=EDGE_CURVE ( 'NONE', #1083, #8633, #8218, .T. ) ;
#5010=DIRECTION ( 'NONE',  ( 0.000000000000000000, 0.000000000000000000, 1.000000000000000000 ) ) ;
#5038=ORIENTED_EDGE ( 'NONE', *, *, #4108, .F. ) ;
#5042=EDGE_LOOP ( 'NONE', ( #6570, #4844, #10127, #2290 ) ) ;
#5045=LINE ( 'NONE', #860, #8595 ) ;
#5046=DIRECTION ( 'NONE',  ( 1.000000000000000000, -0.000000000000000000, -0.000000000000000000 ) ) ;
#5049=CARTESIAN_POINT ( 'NONE',  ( -30.29350689640809335, 2.445795361565304815E-15, 20.00000000000002132 ) ) ;
#5055=ADVANCED_BREP_SHAPE_REPRESENTATION ( '', ( #3077, #4601 ), #9214 ) ;
#5057=ADVANCED_FACE ( 'NONE', ( #7929 ), #2996, .T. ) ;
#5058=VERTEX_POINT ( 'NONE', #5428 ) ;
#5059=AXIS2_PLACEMENT_3D ( 'NONE', #6565, #7415, #8207 ) ;
#5063=FACE_OUTER_BOUND ( 'NONE', #2952, .T. ) ;
#5067=LINE ( 'NONE', #9050, #7736 ) ;
#5071=ORIENTED_EDGE ( 'NONE', *, *, #4977, .F. ) ;
#5084=ADVANCED_FACE ( 'NONE', ( #8236, #7235 ), #5794, .T. ) ;
#5097=VECTOR ( 'NONE', #495, 1000.000000000000000 ) ;
#5100=LINE ( 'NONE', #5787, #1034 ) ;
#5109=VECTOR ( 'NONE', #5881, 1000.000000000000000 ) ;
#5113=ORIENTED_EDGE ( 'NONE', *, *, #2873, .F. ) ;
#5117=DIRECTION ( 'NONE',  ( 0.000000000000000000, 0.000000000000000000, 1.000000000000000000 ) ) ;
#5119=FACE_OUTER_BOUND ( 'NONE', #3288, .T. ) ;
#5120=ORIENTED_EDGE ( 'NONE', *, *, #8198, .F. ) ;
#5126=CARTESIAN_POINT ( 'NONE',  ( -20.29350689640809691, 140.5696653505793563, 19.97500000000000853 ) ) ;
#5133=EDGE_CURVE ( 'NONE', #822, #5783, #5684, .T. ) ;
#5137=DIRECTION ( 'NONE',  ( 0.000000000000000000, 0.000000000000000000, 1.000000000000000000 ) ) ;
#5139=DIRECTION ( 'NONE',  ( -1.000000000000000000, -0.000000000000000000, -0.000000000000000000 ) ) ;
#5143=CARTESIAN_POINT ( 'NONE',  ( -16.29350689640809691, 55.56966535057936341, 0.000000000000000000 ) ) ;
#5150=CARTESIAN_POINT ( 'NONE',  ( -30.29350689640809335, 2.445795361565304815E-15, 20.00000000000002132 ) ) ;
#5162=VERTEX_POINT ( 'NONE', #138 ) ;
#5173=EDGE_CURVE ( 'NONE', #8863, #10023, #1668, .T. ) ;
#5181=DIRECTION ( 'NONE',  ( -0.000000000000000000, 0.000000000000000000, -1.000000000000000000 ) ) ;
#5189=VERTEX_POINT ( 'NONE', #8872 ) ;
#5211=AXIS2_PLACEMENT_3D ( 'NONE', #7067, #7270, #9453 ) ;
#5217=CARTESIAN_POINT ( 'NONE',  ( -2.293506896408097795, 80.56966535057935630, 16.00000000000000711 ) ) ;
#5227=ORIENTED_EDGE ( 'NONE', *, *, #6434, .T. ) ;
#5228=DIRECTION ( 'NONE',  ( 0.000000000000000000, -1.000000000000000000, -1.222897680782651224E-16 ) ) ;
#5239=ORIENTED_EDGE ( 'NONE', *, *, #7737, .T. ) ;
#5251=CARTESIAN_POINT ( 'NONE',  ( -7.293506896408105789, 112.5696653505793705, 20.00000000000000711 ) ) ;
#5252=FACE_OUTER_BOUND ( 'NONE', #8081, .T. ) ;
#5254=DIRECTION ( 'NONE',  ( 0.000000000000000000, 0.000000000000000000, 1.000000000000000000 ) ) ;
#5260=DIRECTION ( 'NONE',  ( 0.000000000000000000, -1.000000000000000000, -1.222897680782651224E-16 ) ) ;
#5276=CARTESIAN_POINT ( 'NONE',  ( -30.29350689640809335, 80.56966535057935630, 20.00000000000000711 ) ) ;
#5284=DIRECTION ( 'NONE',  ( 1.000000000000000000, 0.000000000000000000, 0.000000000000000000 ) ) ;
#5291=CARTESIAN_POINT ( 'NONE',  ( -16.29350689640810756, 140.5696653505793563, 10.98204862120179826 ) ) ;
#5298=ORIENTED_EDGE ( 'NONE', *, *, #2943, .T. ) ;
#5303=DIRECTION ( 'NONE',  ( 0.000000000000000000, 1.000000000000000000, -1.460512169908342690E-16 ) ) ;
#5315=CARTESIAN_POINT ( 'NONE',  ( -30.29350689640809335, 120.5696653505793705, -20.00000000000000711 ) ) ;
#5316=ORIENTED_EDGE ( 'NONE', *, *, #9817, .F. ) ;
#5322=EDGE_LOOP ( 'NONE', ( #1334, #1891, #7324, #4831 ) ) ;
#5331=CARTESIAN_POINT ( 'NONE',  ( -7.293506896408097795, 145.5696653505793563, -20.00000000000000711 ) ) ;
#5338=DIRECTION ( 'NONE',  ( 0.000000000000000000, 0.000000000000000000, 1.000000000000000000 ) ) ;
#5342=DIRECTION ( 'NONE',  ( 0.000000000000000000, 0.000000000000000000, 1.000000000000000000 ) ) ;
#5344=ORIENTED_EDGE ( 'NONE', *, *, #8331, .F. ) ;
#5355=VECTOR ( 'NONE', #8036, 1000.000000000000000 ) ;
#5371=EDGE_CURVE ( 'NONE', #3083, #8958, #3896, .T. ) ;
#5373=AXIS2_PLACEMENT_3D ( 'NONE', #4138, #8216, #8110 ) ;
#5377=EDGE_LOOP ( 'NONE', ( #7066, #8281 ) ) ;
#5378=DIRECTION ( 'NONE',  ( 0.000000000000000000, 0.000000000000000000, -1.000000000000000000 ) ) ;
#5379=ORIENTED_EDGE ( 'NONE', *, *, #1140, .F. ) ;
#5389=CYLINDRICAL_SURFACE ( 'NONE', #7573, 7.999999999999989342 ) ;
#5391=DIRECTION ( 'NONE',  ( 0.000000000000000000, 0.000000000000000000, -1.000000000000000000 ) ) ;
#5396=ORIENTED_EDGE ( 'NONE', *, *, #6053, .F. ) ;
#5401=DIRECTION ( 'NONE',  ( 1.000000000000000000, -0.000000000000000000, -0.000000000000000000 ) ) ;
#5421=ADVANCED_FACE ( 'NONE', ( #2244 ), #8706, .T. ) ;
#5422=ORIENTED_EDGE ( 'NONE', *, *, #9951, .T. ) ;
#5423=CARTESIAN_POINT ( 'NONE',  ( -2.293506896408097795, 37.08684478514406635, 15.00000000000000355 ) ) ;
#5427=DIRECTION ( 'NONE',  ( 1.000000000000000000, 0.000000000000000000, 0.000000000000000000 ) ) ;
#5428=CARTESIAN_POINT ( 'NONE',  ( -7.293506896408097795, 72.56966535057935630, -20.00000000000001066 ) ) ;
#5429=VERTEX_POINT ( 'NONE', #9400 ) ;
#5436=ORIENTED_EDGE ( 'NONE', *, *, #10263, .T. ) ;
#5448=VECTOR ( 'NONE', #7856, 1000.000000000000000 ) ;
#5449=ORIENTED_EDGE ( 'NONE', *, *, #2399, .T. ) ;
#5451=ORIENTED_EDGE ( 'NONE', *, *, #9615, .T. ) ;
#5461=VERTEX_POINT ( 'NONE', #6371 ) ;
#5465=ORIENTED_EDGE ( 'NONE', *, *, #6506, .T. ) ;
#5466=VERTEX_POINT ( 'NONE', #3239 ) ;
#5468=CARTESIAN_POINT ( 'NONE',  ( -24.29350689640808625, 140.5696653505793563, -20.00000000000000711 ) ) ;
#5469=CARTESIAN_POINT ( 'NONE',  ( -30.29350689640809335, 2.445795361565304815E-15, -20.00000000000002132 ) ) ;
#5470=CARTESIAN_POINT ( 'NONE',  ( -16.29350689640810756, 140.5696653505793563, 20.00000000000002132 ) ) ;
#5471=EDGE_CURVE ( 'NONE', #510, #3403, #8862, .T. ) ;
#5500=ORIENTED_EDGE ( 'NONE', *, *, #4093, .F. ) ;
#5511=VECTOR ( 'NONE', #5046, 1000.000000000000000 ) ;
#5526=CIRCLE ( 'NONE', #10287, 3.999999999999989786 ) ;
#5543=EDGE_CURVE ( 'NONE', #4361, #39, #4981, .T. ) ;
#5544=EDGE_CURVE ( 'NONE', #2948, #6365, #4880, .T. ) ;
#5551=FACE_OUTER_BOUND ( 'NONE', #8697, .T. ) ;
#5556=VERTEX_POINT ( 'NONE', #2446 ) ;
#5561=CARTESIAN_POINT ( 'NONE',  ( -30.29350689640809335, 150.5696653505793563, -20.00000000000000355 ) ) ;
#5566=DIRECTION ( 'NONE',  ( -1.000000000000000000, -0.000000000000000000, -0.000000000000000000 ) ) ;
#5575=CARTESIAN_POINT ( 'NONE',  ( -30.29350689640809335, 120.5696653505793705, 20.00000000000000711 ) ) ;
#5577=VERTEX_POINT ( 'NONE', #8166 ) ;
#5590=CARTESIAN_POINT ( 'NONE',  ( -20.29350689640809691, 140.5696653505793563, -10.98204862120179826 ) ) ;
#5592=ORIENTED_EDGE ( 'NONE', *, *, #1198, .T. ) ;
#5594=VECTOR ( 'NONE', #3918, 1000.000000000000000 ) ;
#5595=CYLINDRICAL_SURFACE ( 'NONE', #5986, 10.00000000000000000 ) ;
#5598=CYLINDRICAL_SURFACE ( 'NONE', #3475, 4.000000000000000000 ) ;
#5599=EDGE_CURVE ( 'NONE', #8767, #1043, #9124, .T. ) ;
#5606=ORIENTED_EDGE ( 'NONE', *, *, #10408, .F. ) ;
#5614=ORIENTED_EDGE ( 'NONE', *, *, #9010, .F. ) ;
#5622=LINE ( 'NONE', #7220, #7665 ) ;
#5634=DIRECTION ( 'NONE',  ( 0.000000000000000000, 0.000000000000000000, -1.000000000000000000 ) ) ;
#5635=EDGE_LOOP ( 'NONE', ( #5113, #3181, #4344, #3407, #2519 ) ) ;
#5642=ORIENTED_EDGE ( 'NONE', *, *, #7364, .T. ) ;
#5645=FACE_BOUND ( 'NONE', #5666, .T. ) ;
#5653=EDGE_CURVE ( 'NONE', #5715, #852, #1015, .T. ) ;
#5656=CARTESIAN_POINT ( 'NONE',  ( -30.29350689640809335, 140.5696653505793563, 20.00000000000000355 ) ) ;
#5659=CARTESIAN_POINT ( 'NONE',  ( -30.29350689640809335, 72.56966535057935630, -20.00000000000001066 ) ) ;
#5660=CARTESIAN_POINT ( 'NONE',  ( 14.70649310359190309, 80.56966535057935630, 24.00000000000000711 ) ) ;
#5665=ORIENTED_EDGE ( 'NONE', *, *, #8390, .T. ) ;
#5666=EDGE_LOOP ( 'NONE', ( #7500, #2457 ) ) ;
#5668=PLANE ( 'NONE',  #7751 ) ;
#5670=FACE_OUTER_BOUND ( 'NONE', #6688, .T. ) ;
#5672=CARTESIAN_POINT ( 'NONE',  ( -7.293506896408097795, 2.445795361565304815E-15, 20.00000000000002132 ) ) ;
#5673=ORIENTED_EDGE ( 'NONE', *, *, #10408, .T. ) ;
#5679=VECTOR ( 'NONE', #8728, 1000.000000000000000 ) ;
#5683=ADVANCED_FACE ( 'NONE', ( #1911 ), #5830, .T. ) ;
#5684=LINE ( 'NONE', #2513, #780 ) ;
#5696=DIRECTION ( 'NONE',  ( 0.000000000000000000, 0.000000000000000000, -1.000000000000000000 ) ) ;
#5705=CARTESIAN_POINT ( 'NONE',  ( -7.293506896408097795, 120.5696653505793705, -20.00000000000000711 ) ) ;
#5710=AXIS2_PLACEMENT_3D ( 'NONE', #5150, #4362, #7598 ) ;
#5711=DIRECTION ( 'NONE',  ( -0.000000000000000000, -0.000000000000000000, 1.000000000000000000 ) ) ;
#5713=EDGE_CURVE ( 'NONE', #195, #1043, #124, .T. ) ;
#5715=VERTEX_POINT ( 'NONE', #2962 ) ;
#5730=VERTEX_POINT ( 'NONE', #3919 ) ;
#5738=EDGE_CURVE ( 'NONE', #4025, #4617, #2274, .T. ) ;
#5746=SHAPE_REPRESENTATION_RELATIONSHIP ( 'NONE' , 'NONE' ,  #6561, #5055 ) ;
#5748=FACE_OUTER_BOUND ( 'NONE', #7341, .T. ) ;
#5753=DIRECTION ( 'NONE',  ( -1.000000000000000000, 0.000000000000000000, 0.000000000000000000 ) ) ;
#5762=ORIENTED_EDGE ( 'NONE', *, *, #1322, .F. ) ;
#5772=LINE ( 'NONE', #6626, #4783 ) ;
#5773=FACE_OUTER_BOUND ( 'NONE', #10137, .T. ) ;
#5777=CARTESIAN_POINT ( 'NONE',  ( -30.29350689640809335, 80.56966535057935630, 20.00000000000000711 ) ) ;
#5783=VERTEX_POINT ( 'NONE', #3814 ) ;
#5784=EDGE_CURVE ( 'NONE', #852, #2923, #1131, .T. ) ;
#5787=CARTESIAN_POINT ( 'NONE',  ( -24.29350689640808625, 140.5696653505793563, 20.00000000000002132 ) ) ;
#5789=LINE ( 'NONE', #9786, #9594 ) ;
#5794=PLANE ( 'NONE',  #8744 ) ;
#5803=FACE_OUTER_BOUND ( 'NONE', #1632, .T. ) ;
#5807=CARTESIAN_POINT ( 'NONE',  ( -20.29350689640809691, 150.5696653505793563, 20.00000000000000355 ) ) ;
#5808=PLANE ( 'NONE',  #6807 ) ;
#5810=FACE_OUTER_BOUND ( 'NONE', #203, .T. ) ;
#5820=ADVANCED_FACE ( 'NONE', ( #4020 ), #7891, .F. ) ;
#5821=ORIENTED_EDGE ( 'NONE', *, *, #731, .F. ) ;
#5830=PLANE ( 'NONE',  #3335 ) ;
#5843=AXIS2_PLACEMENT_3D ( 'NONE', #5907, #8350, #458 ) ;
#5844=ORIENTED_EDGE ( 'NONE', *, *, #7806, .F. ) ;
#5856=AXIS2_PLACEMENT_3D ( 'NONE', #10250, #1183, #2189 ) ;
#5862=VECTOR ( 'NONE', #782, 1000.000000000000000 ) ;
#5863=VERTEX_POINT ( 'NONE', #6293 ) ;
#5867=CIRCLE ( 'NONE', #3846, 4.000000000000000000 ) ;
#5868=CARTESIAN_POINT ( 'NONE',  ( -30.29350689640809335, -0.3998014571812398832, -1.076388538564875708 ) ) ;
#5872=EDGE_CURVE ( 'NONE', #2948, #6283, #1152, .T. ) ;
#5873=ORIENTED_EDGE ( 'NONE', *, *, #2808, .F. ) ;
#5874=ORIENTED_EDGE ( 'NONE', *, *, #5738, .T. ) ;
#5877=ORIENTED_EDGE ( 'NONE', *, *, #4240, .T. ) ;
#5881=DIRECTION ( 'NONE',  ( 0.000000000000000000, 1.000000000000000000, 1.460512169908342690E-16 ) ) ;
#5884=LINE ( 'NONE', #224, #10122 ) ;
#5885=ORIENTED_EDGE ( 'NONE', *, *, #5006, .T. ) ;
#5894=DIRECTION ( 'NONE',  ( 0.000000000000000000, -1.000000000000000000, -1.222897680782651471E-16 ) ) ;
#5907=CARTESIAN_POINT ( 'NONE',  ( 14.70649310359190309, 80.56966535057935630, 20.00000000000000711 ) ) ;
#5909=EDGE_CURVE ( 'NONE', #4261, #954, #2580, .T. ) ;
#5913=FACE_OUTER_BOUND ( 'NONE', #2590, .T. ) ;
#5917=CARTESIAN_POINT ( 'NONE',  ( -20.29350689640809691, 140.5696653505793563, 20.00000000000002132 ) ) ;
#5923=CARTESIAN_POINT ( 'NONE',  ( -30.29350689640809335, 112.5696653505793705, -20.00000000000000711 ) ) ;
#5925=VERTEX_POINT ( 'NONE', #9962 ) ;
#5928=DIRECTION ( 'NONE',  ( 1.000000000000000000, 0.000000000000000000, 0.000000000000000000 ) ) ;
#5949=ADVANCED_FACE ( 'NONE', ( #1784 ), #5808, .T. ) ;
#5952=ORIENTED_EDGE ( 'NONE', *, *, #5599, .T. ) ;
#5969=ORIENTED_EDGE ( 'NONE', *, *, #7672, .T. ) ;
#5971=CARTESIAN_POINT ( 'NONE',  ( -7.293506896408105789, 128.5696653505793563, -20.00000000000000711 ) ) ;
#5974=CARTESIAN_POINT ( 'NONE',  ( -16.29350689640809691, 37.08684478514406635, 0.000000000000000000 ) ) ;
#5979=VECTOR ( 'NONE', #8208, 1000.000000000000000 ) ;
#5983=DIRECTION ( 'NONE',  ( 0.000000000000000000, 0.000000000000000000, 1.000000000000000000 ) ) ;
#5986=AXIS2_PLACEMENT_3D ( 'NONE', #6394, #4704, #10379 ) ;
#5996=CARTESIAN_POINT ( 'NONE',  ( -7.293506896408097795, 4.007378841484243628E-15, -28.00000000000002132 ) ) ;
#6005=DIRECTION ( 'NONE',  ( 1.000000000000000000, -0.000000000000000000, -0.000000000000000000 ) ) ;
#6023=CIRCLE ( 'NONE', #9774, 7.999999999999996447 ) ;
#6053=EDGE_CURVE ( 'NONE', #7959, #8633, #9203, .T. ) ;
#6054=EDGE_CURVE ( 'NONE', #1695, #4328, #4449, .T. ) ;
#6058=ORIENTED_EDGE ( 'NONE', *, *, #6932, .T. ) ;
#6060=CIRCLE ( 'NONE', #1501, 10.00000000000000178 ) ;
#6061=CARTESIAN_POINT ( 'NONE',  ( -7.293506896408097795, 2.445795361565304815E-15, -20.00000000000002132 ) ) ;
#6062=VECTOR ( 'NONE', #432, 1000.000000000000000 ) ;
#6068=DIRECTION ( 'NONE',  ( -1.000000000000000000, 0.000000000000000000, 0.000000000000000000 ) ) ;
#6072=VERTEX_POINT ( 'NONE', #7715 ) ;
#6085=VERTEX_POINT ( 'NONE', #3743 ) ;
#6089=ORIENTED_EDGE ( 'NONE', *, *, #1831, .T. ) ;
#6116=CARTESIAN_POINT ( 'NONE',  ( -16.29350689640809691, 37.08684478514406635, -7.500000000000000000 ) ) ;
#6123=ORIENTED_EDGE ( 'NONE', *, *, #10339, .T. ) ;
#6127=VECTOR ( 'NONE', #938, 1000.000000000000000 ) ;
#6135=DIRECTION ( 'NONE',  ( -0.000000000000000000, -1.000000000000000000, -0.000000000000000000 ) ) ;
#6146=EDGE_CURVE ( 'NONE', #3604, #1079, #9532, .T. ) ;
#6159=ADVANCED_FACE ( 'NONE', ( #3202 ), #7030, .F. ) ;
#6164=AXIS2_PLACEMENT_3D ( 'NONE', #6883, #5181, #2004 ) ;
#6176=ORIENTED_EDGE ( 'NONE', *, *, #6662, .T. ) ;
#6180=ORIENTED_EDGE ( 'NONE', *, *, #7032, .T. ) ;
#6189=ADVANCED_FACE ( 'NONE', ( #8721 ), #7875, .F. ) ;
#6192=AXIS2_PLACEMENT_3D ( 'NONE', #8371, #7296, #3214 ) ;
#6199=ORIENTED_EDGE ( 'NONE', *, *, #5543, .F. ) ;
#6211=FACE_BOUND ( 'NONE', #7995, .T. ) ;
#6226=CARTESIAN_POINT ( 'NONE',  ( -7.293506896408097795, 0.000000000000000000, 0.000000000000000000 ) ) ;
#6237=DIRECTION ( 'NONE',  ( -1.000000000000000000, 0.000000000000000000, 0.000000000000000000 ) ) ;
#6242=CARTESIAN_POINT ( 'NONE',  ( 0.000000000000000000, 55.56966535057937051, -10.98204862120179826 ) ) ;
#6260=ORIENTED_EDGE ( 'NONE', *, *, #4501, .T. ) ;
#6262=EDGE_LOOP ( 'NONE', ( #9221, #4056, #10191, #1205 ) ) ;
#6275=DIRECTION ( 'NONE',  ( -0.000000000000000000, -0.000000000000000000, -1.000000000000000000 ) ) ;
#6283=VERTEX_POINT ( 'NONE', #6596 ) ;
#6284=AXIS2_PLACEMENT_3D ( 'NONE', #6752, #10151, #6859 ) ;
#6293=CARTESIAN_POINT ( 'NONE',  ( -2.293506896408097795, 145.5696653505793563, 25.00000000000000711 ) ) ;
#6301=CYLINDRICAL_SURFACE ( 'NONE', #9338, 7.999999999999996447 ) ;
#6314=AXIS2_PLACEMENT_3D ( 'NONE', #3967, #7250, #6349 ) ;
#6315=ORIENTED_EDGE ( 'NONE', *, *, #6054, .T. ) ;
#6328=CIRCLE ( 'NONE', #9717, 3.999999999999989786 ) ;
#6332=CARTESIAN_POINT ( 'NONE',  ( -30.29350689640809335, 37.08684478514406635, 15.00000000000000355 ) ) ;
#6338=ORIENTED_EDGE ( 'NONE', *, *, #3494, .T. ) ;
#6342=AXIS2_PLACEMENT_3D ( 'NONE', #2885, #9358, #10319 ) ;
#6347=CARTESIAN_POINT ( 'NONE',  ( -2.293506896408101348, 150.5696653505793563, 10.98204862120179826 ) ) ;
#6349=DIRECTION ( 'NONE',  ( 1.000000000000000000, 0.000000000000000000, 0.000000000000000000 ) ) ;
#6356=VERTEX_POINT ( 'NONE', #7447 ) ;
#6357=CARTESIAN_POINT ( 'NONE',  ( -30.29350689640809335, 150.5696653505793563, 20.00000000000000711 ) ) ;
#6361=VERTEX_POINT ( 'NONE', #190 ) ;
#6362=VERTEX_POINT ( 'NONE', #9732 ) ;
#6365=VERTEX_POINT ( 'NONE', #2516 ) ;
#6371=CARTESIAN_POINT ( 'NONE',  ( -30.29350689640809335, 55.56966535057937051, 10.98204862120179826 ) ) ;
#6376=ORIENTED_EDGE ( 'NONE', *, *, #3787, .T. ) ;
#6382=LINE ( 'NONE', #7769, #10258 ) ;
#6386=VECTOR ( 'NONE', #67, 1000.000000000000000 ) ;
#6394=CARTESIAN_POINT ( 'NONE',  ( -20.29350689640809691, 140.5696653505793563, 0.000000000000000000 ) ) ;
#6396=LINE ( 'NONE', #3061, #4583 ) ;
#6399=EDGE_LOOP ( 'NONE', ( #843, #5673, #4402, #9258, #3643 ) ) ;
#6409=VECTOR ( 'NONE', #5260, 1000.000000000000000 ) ;
#6413=ORIENTED_EDGE ( 'NONE', *, *, #7577, .F. ) ;
#6416=DIRECTION ( 'NONE',  ( 0.000000000000000000, 1.000000000000000000, 0.000000000000000000 ) ) ;
#6434=EDGE_CURVE ( 'NONE', #1117, #4058, #1080, .T. ) ;
#6436=CYLINDRICAL_SURFACE ( 'NONE', #2679, 5.000000000000000888 ) ;
#6443=DIRECTION ( 'NONE',  ( 1.000000000000000000, -0.000000000000000000, -0.000000000000000000 ) ) ;
#6463=AXIS2_PLACEMENT_3D ( 'NONE', #5917, #2899, #1102 ) ;
#6469=LINE ( 'NONE', #5470, #8501 ) ;
#6472=VECTOR ( 'NONE', #7018, 1000.000000000000000 ) ;
#6473=ORIENTED_EDGE ( 'NONE', *, *, #1683, .T. ) ;
#6482=DIRECTION ( 'NONE',  ( 0.000000000000000000, 0.000000000000000000, 1.000000000000000000 ) ) ;
#6484=VERTEX_POINT ( 'NONE', #7705 ) ;
#6490=VERTEX_POINT ( 'NONE', #6915 ) ;
#6498=LINE ( 'NONE', #5807, #9851 ) ;
#6503=VECTOR ( 'NONE', #522, 1000.000000000000000 ) ;
#6506=EDGE_CURVE ( 'NONE', #8244, #1695, #8847, .T. ) ;
#6507=DIRECTION ( 'NONE',  ( 1.000000000000000000, -0.000000000000000000, -0.000000000000000000 ) ) ;
#6512=AXIS2_PLACEMENT_3D ( 'NONE', #2230, #5711, #1898 ) ;
#6517=ORIENTED_EDGE ( 'NONE', *, *, #1669, .F. ) ;
#6525=CARTESIAN_POINT ( 'NONE',  ( -2.293506896408097795, -0.3998014571812398832, 1.076388538564875708 ) ) ;
#6534=DIRECTION ( 'NONE',  ( 0.000000000000000000, -1.000000000000000000, 0.000000000000000000 ) ) ;
#6535=CARTESIAN_POINT ( 'NONE',  ( 67.68113203623319407, 150.5696653505793563, 10.98204862120179826 ) ) ;
#6544=VECTOR ( 'NONE', #2026, 1000.000000000000000 ) ;
#6546=DIRECTION ( 'NONE',  ( 0.000000000000000000, 0.000000000000000000, -1.000000000000000000 ) ) ;
#6548=EDGE_LOOP ( 'NONE', ( #1556, #6764, #8105, #5500 ) ) ;
#6561=SHAPE_REPRESENTATION ( 'Metal Mounting Block', ( #4601 ), #9214 ) ;
#6564=DIRECTION ( 'NONE',  ( 0.000000000000000000, 1.734723475976809067E-15, 1.000000000000000000 ) ) ;
#6565=CARTESIAN_POINT ( 'NONE',  ( -2.293506896408097795, 80.56966535057935630, -20.00000000000000711 ) ) ;
#6570=ORIENTED_EDGE ( 'NONE', *, *, #8842, .F. ) ;
#6579=CARTESIAN_POINT ( 'NONE',  ( 67.68113203623319407, 65.56966535057937051, 10.98204862120179826 ) ) ;
#6591=DIRECTION ( 'NONE',  ( 1.000000000000000000, -0.000000000000000000, -0.000000000000000000 ) ) ;
#6594=CARTESIAN_POINT ( 'NONE',  ( -30.29350689640809335, 37.08684478514406635, 0.000000000000000000 ) ) ;
#6596=CARTESIAN_POINT ( 'NONE',  ( -30.29350689640809335, 80.56966535057935630, -24.00000000000000711 ) ) ;
#6623=CARTESIAN_POINT ( 'NONE',  ( -2.293506896408097795, -3.651280424770854409E-15, 24.99999999999998579 ) ) ;
#6626=CARTESIAN_POINT ( 'NONE',  ( -30.29350689640809335, 2.445795361565304815E-15, 20.00000000000002132 ) ) ;
#6630=EDGE_CURVE ( 'NONE', #6085, #6356, #9402, .T. ) ;
#6639=DIRECTION ( 'NONE',  ( 1.000000000000000000, -0.000000000000000000, -0.000000000000000000 ) ) ;
#6646=CARTESIAN_POINT ( 'NONE',  ( -24.29350689640808625, 140.5696653505793563, 10.98204862120179826 ) ) ;
#6656=CARTESIAN_POINT ( 'NONE',  ( -30.29350689640809335, 2.445795361565304815E-15, -20.00000000000002132 ) ) ;
#6662=EDGE_CURVE ( 'NONE', #5577, #4058, #3758, .T. ) ;
#6663=VERTEX_POINT ( 'NONE', #3091 ) ;
#6664=DIRECTION ( 'NONE',  ( 0.000000000000000000, -0.3481865296036273372, 0.9374252720097653313 ) ) ;
#6667=DIRECTION ( 'NONE',  ( 1.000000000000000000, -0.000000000000000000, -0.000000000000000000 ) ) ;
#6672=DIRECTION ( 'NONE',  ( 1.000000000000000000, -0.000000000000000000, -0.000000000000000000 ) ) ;
#6674=ORIENTED_EDGE ( 'NONE', *, *, #7719, .T. ) ;
#6681=DIRECTION ( 'NONE',  ( -1.000000000000000000, 0.000000000000000000, 0.000000000000000000 ) ) ;
#6688=EDGE_LOOP ( 'NONE', ( #1295, #6338, #2043, #2447 ) ) ;
#6701=VECTOR ( 'NONE', #1206, 1000.000000000000000 ) ;
#6703=DIRECTION ( 'NONE',  ( 1.000000000000000000, -0.000000000000000000, -0.000000000000000000 ) ) ;
#6707=FACE_OUTER_BOUND ( 'NONE', #3959, .T. ) ;
#6725=AXIS2_PLACEMENT_3D ( 'NONE', #2398, #9576, #8071 ) ;
#6736=DIRECTION ( 'NONE',  ( 0.000000000000000000, 0.000000000000000000, 1.000000000000000000 ) ) ;
#6737=EDGE_LOOP ( 'NONE', ( #99, #6892, #1109, #8343 ) ) ;
#6745=LINE ( 'NONE', #7440, #5511 ) ;
#6748=EDGE_CURVE ( 'NONE', #5730, #596, #8485, .T. ) ;
#6752=CARTESIAN_POINT ( 'NONE',  ( -30.29350689640809335, 80.56966535057935630, -20.00000000000000711 ) ) ;
#6757=DIRECTION ( 'NONE',  ( 0.000000000000000000, 0.000000000000000000, -1.000000000000000000 ) ) ;
#6764=ORIENTED_EDGE ( 'NONE', *, *, #3194, .T. ) ;
#6772=CARTESIAN_POINT ( 'NONE',  ( -2.293506896408097795, 0.000000000000000000, -10.98204862120179826 ) ) ;
#6773=PRODUCT_DEFINITION ( 'UNKNOWN', '', #4471, #1020 ) ;
#6804=EDGE_CURVE ( 'NONE', #2451, #288, #10237, .T. ) ;
#6807=AXIS2_PLACEMENT_3D ( 'NONE', #7353, #153, #5010 ) ;
#6808=CARTESIAN_POINT ( 'NONE',  ( -20.29350689640810046, 150.5696653505793563, 20.00000000000000355 ) ) ;
#6813=DIRECTION ( 'NONE',  ( 0.000000000000000000, -1.000000000000000000, 0.000000000000000000 ) ) ;
#6819=ADVANCED_FACE ( 'NONE', ( #8689 ), #6301, .T. ) ;
#6829=LINE ( 'NONE', #6939, #6503 ) ;
#6834=CARTESIAN_POINT ( 'NONE',  ( -30.29350689640809335, 120.5696653505793705, -20.00000000000000711 ) ) ;
#6838=LINE ( 'NONE', #7527, #6062 ) ;
#6842=CARTESIAN_POINT ( 'NONE',  ( -2.293506896408097795, 120.5696653505793705, 16.00000000000000711 ) ) ;
#6855=ADVANCED_FACE ( 'NONE', ( #209 ), #10478, .T. ) ;
#6859=DIRECTION ( 'NONE',  ( 0.000000000000000000, 0.000000000000000000, 1.000000000000000000 ) ) ;
#6861=LINE ( 'NONE', #8554, #2352 ) ;
#6864=CYLINDRICAL_SURFACE ( 'NONE', #1814, 7.999999999999994671 ) ;
#6875=DIRECTION ( 'NONE',  ( 1.000000000000000000, -0.000000000000000000, -0.000000000000000000 ) ) ;
#6883=CARTESIAN_POINT ( 'NONE',  ( 67.68113203623319407, 65.56966535057937051, -10.98204862120179826 ) ) ;
#6892=ORIENTED_EDGE ( 'NONE', *, *, #8084, .F. ) ;
#6897=ORIENTED_EDGE ( 'NONE', *, *, #4977, .T. ) ;
#6914=ORIENTED_EDGE ( 'NONE', *, *, #3925, .T. ) ;
#6915=CARTESIAN_POINT ( 'NONE',  ( -30.29350689640809335, 55.56966535057937051, -10.98204862120179826 ) ) ;
#6932=EDGE_CURVE ( 'NONE', #6072, #6943, #2055, .T. ) ;
#6933=VERTEX_POINT ( 'NONE', #7258 ) ;
#6939=CARTESIAN_POINT ( 'NONE',  ( 14.70649310359190309, 80.56966535057935630, 16.00000000000000711 ) ) ;
#6943=VERTEX_POINT ( 'NONE', #7414 ) ;
#6952=ORIENTED_EDGE ( 'NONE', *, *, #3494, .F. ) ;
#6960=AXIS2_PLACEMENT_3D ( 'NONE', #1624, #9801, #3270 ) ;
#6967=ADVANCED_FACE ( 'NONE', ( #7306 ), #51, .F. ) ;
#6972=CARTESIAN_POINT ( 'NONE',  ( -16.26850689640809478, 140.5696653505793563, 20.00000000000002132 ) ) ;
#6975=DIRECTION ( 'NONE',  ( 0.000000000000000000, 0.000000000000000000, 1.000000000000000000 ) ) ;
#6976=ORIENTED_EDGE ( 'NONE', *, *, #2547, .T. ) ;
#6982=AXIS2_PLACEMENT_3D ( 'NONE', #10323, #7138, #5378 ) ;
#7001=CARTESIAN_POINT ( 'NONE',  ( -2.293506896408097795, 4.007378841484243628E-15, -28.00000000000002132 ) ) ;
#7006=DIRECTION ( 'NONE',  ( 0.000000000000000000, 1.222897680782651471E-16, 1.000000000000000000 ) ) ;
#7010=EDGE_CURVE ( 'NONE', #6356, #6484, #3547, .T. ) ;
#7012=ORIENTED_EDGE ( 'NONE', *, *, #2125, .F. ) ;
#7018=DIRECTION ( 'NONE',  ( 0.000000000000000000, -1.000000000000000000, 1.222897680782651224E-16 ) ) ;
#7022=EDGE_CURVE ( 'NONE', #8863, #39, #4282, .T. ) ;
#7026=DIRECTION ( 'NONE',  ( 0.000000000000000000, 1.000000000000000000, -1.460512169908342690E-16 ) ) ;
#7030=PLANE ( 'NONE',  #6982 ) ;
#7032=EDGE_CURVE ( 'NONE', #8054, #5162, #7726, .T. ) ;
#7037=CARTESIAN_POINT ( 'NONE',  ( -30.29350689640809335, 88.56966535057934209, -20.00000000000001066 ) ) ;
#7040=DIRECTION ( 'NONE',  ( 0.000000000000000000, -1.000000000000000000, 1.222897680782651471E-16 ) ) ;
#7054=VERTEX_POINT ( 'NONE', #1844 ) ;
#7064=AXIS2_PLACEMENT_3D ( 'NONE', #579, #1481, #633 ) ;
#7066=ORIENTED_EDGE ( 'NONE', *, *, #8828, .F. ) ;
#7067=CARTESIAN_POINT ( 'NONE',  ( -2.293506896408097795, 0.000000000000000000, 0.000000000000000000 ) ) ;
#7079=VECTOR ( 'NONE', #5566, 1000.000000000000000 ) ;
#7086=DIRECTION ( 'NONE',  ( -1.000000000000000000, 0.000000000000000000, 0.000000000000000000 ) ) ;
#7089=VERTEX_POINT ( 'NONE', #5971 ) ;
#7095=ADVANCED_FACE ( 'NONE', ( #8361 ), #8158, .F. ) ;
#7106=DIRECTION ( 'NONE',  ( -1.000000000000000000, 0.000000000000000000, 0.000000000000000000 ) ) ;
#7133=LINE ( 'NONE', #4088, #4688 ) ;
#7138=DIRECTION ( 'NONE',  ( 0.000000000000000000, -1.000000000000000000, -0.000000000000000000 ) ) ;
#7172=CARTESIAN_POINT ( 'NONE',  ( -7.293506896408097795, 145.5696653505793563, 25.00000000000000711 ) ) ;
#7174=CIRCLE ( 'NONE', #2419, 5.000000000000000888 ) ;
#7185=AXIS2_PLACEMENT_3D ( 'NONE', #7505, #8404, #7558 ) ;
#7188=CARTESIAN_POINT ( 'NONE',  ( -30.29350689640809335, 120.5696653505793705, 24.00000000000000711 ) ) ;
#7213=ORIENTED_EDGE ( 'NONE', *, *, #2219, .F. ) ;
#7217=CARTESIAN_POINT ( 'NONE',  ( -7.293506896408097795, 80.56966535057935630, 28.00000000000001066 ) ) ;
#7220=CARTESIAN_POINT ( 'NONE',  ( 0.000000000000000000, 55.56966535057937051, 10.98204862120179826 ) ) ;
#7222=EDGE_CURVE ( 'NONE', #852, #10322, #2158, .T. ) ;
#7228=VECTOR ( 'NONE', #6875, 1000.000000000000000 ) ;
#7234=DIRECTION ( 'NONE',  ( -1.000000000000000000, 0.000000000000000000, 0.000000000000000000 ) ) ;
#7235=FACE_OUTER_BOUND ( 'NONE', #4740, .T. ) ;
#7239=AXIS2_PLACEMENT_3D ( 'NONE', #4922, #3397, #8277 ) ;
#7248=FACE_OUTER_BOUND ( 'NONE', #1788, .T. ) ;
#7250=DIRECTION ( 'NONE',  ( -0.000000000000000000, -0.000000000000000000, 1.000000000000000000 ) ) ;
#7255=ORIENTED_EDGE ( 'NONE', *, *, #5371, .F. ) ;
#7257=CARTESIAN_POINT ( 'NONE',  ( -30.29350689640809335, 120.5696653505793705, 16.00000000000000711 ) ) ;
#7258=CARTESIAN_POINT ( 'NONE',  ( -30.29350689640809335, 120.5696653505793705, -27.99999999999999645 ) ) ;
#7270=DIRECTION ( 'NONE',  ( -1.000000000000000000, 0.000000000000000000, 0.000000000000000000 ) ) ;
#7278=EDGE_CURVE ( 'NONE', #2007, #4617, #9945, .T. ) ;
#7282=DIRECTION ( 'NONE',  ( 1.000000000000000000, 0.000000000000000000, 0.000000000000000000 ) ) ;
#7296=DIRECTION ( 'NONE',  ( -0.000000000000000000, -0.000000000000000000, 1.000000000000000000 ) ) ;
#7306=FACE_OUTER_BOUND ( 'NONE', #410, .T. ) ;
#7315=ORIENTED_EDGE ( 'NONE', *, *, #8775, .F. ) ;
#7323=CARTESIAN_POINT ( 'NONE',  ( -24.31850689640809549, 140.5696653505793563, 20.00000000000002132 ) ) ;
#7324=ORIENTED_EDGE ( 'NONE', *, *, #9537, .F. ) ;
#7329=VECTOR ( 'NONE', #398, 1000.000000000000000 ) ;
#7341=EDGE_LOOP ( 'NONE', ( #2598, #9072, #966, #1838, #1804 ) ) ;
#7353=CARTESIAN_POINT ( 'NONE',  ( -7.293506896408097795, 0.000000000000000000, 0.000000000000000000 ) ) ;
#7364=EDGE_CURVE ( 'NONE', #4025, #5863, #2921, .T. ) ;
#7372=EDGE_LOOP ( 'NONE', ( #5844, #9698, #2770, #4792 ) ) ;
#7375=ORIENTED_EDGE ( 'NONE', *, *, #3194, .F. ) ;
#7377=AXIS2_PLACEMENT_3D ( 'NONE', #5126, #8360, #469 ) ;
#7400=DIRECTION ( 'NONE',  ( 0.000000000000000000, 0.000000000000000000, 1.000000000000000000 ) ) ;
#7412=EDGE_LOOP ( 'NONE', ( #9174, #8854 ) ) ;
#7413=DIRECTION ( 'NONE',  ( -1.000000000000000000, 0.000000000000000000, 0.000000000000000000 ) ) ;
#7414=CARTESIAN_POINT ( 'NONE',  ( -2.293506896408097795, 126.8146633489777599, -25.00000000000000000 ) ) ;
#7415=DIRECTION ( 'NONE',  ( 1.000000000000000000, -0.000000000000000000, -0.000000000000000000 ) ) ;
#7424=AXIS2_PLACEMENT_3D ( 'NONE', #3384, #7413, #4071 ) ;
#7429=VECTOR ( 'NONE', #855, 1000.000000000000114 ) ;
#7434=LINE ( 'NONE', #9021, #7429 ) ;
#7436=ORIENTED_EDGE ( 'NONE', *, *, #6506, .F. ) ;
#7440=CARTESIAN_POINT ( 'NONE',  ( -30.29350689640809335, 72.56966535057935630, 20.00000000000001066 ) ) ;
#7447=CARTESIAN_POINT ( 'NONE',  ( -7.293506896408097795, 80.56966535057935630, -28.00000000000001066 ) ) ;
#7469=AXIS2_PLACEMENT_3D ( 'NONE', #4327, #6068, #1937 ) ;
#7470=EDGE_LOOP ( 'NONE', ( #10111, #9232 ) ) ;
#7473=DIRECTION ( 'NONE',  ( 0.000000000000000000, 0.000000000000000000, 1.000000000000000000 ) ) ;
#7483=EDGE_CURVE ( 'NONE', #1439, #8633, #8651, .T. ) ;
#7485=CARTESIAN_POINT ( 'NONE',  ( -2.293506896408101348, 150.5696653505793563, -10.98204862120179826 ) ) ;
#7500=ORIENTED_EDGE ( 'NONE', *, *, #7765, .F. ) ;
#7503=EDGE_LOOP ( 'NONE', ( #5614, #2058, #10115, #2127 ) ) ;
#7504=CARTESIAN_POINT ( 'NONE',  ( -30.29350689640809335, 80.56966535057935630, 24.00000000000000711 ) ) ;
#7505=CARTESIAN_POINT ( 'NONE',  ( -30.29350689640809335, 120.5696653505793705, 20.00000000000000711 ) ) ;
#7513=EDGE_CURVE ( 'NONE', #13, #2019, #4453, .T. ) ;
#7518=LINE ( 'NONE', #5868, #8011 ) ;
#7525=ORIENTED_EDGE ( 'NONE', *, *, #5544, .T. ) ;
#7527=CARTESIAN_POINT ( 'NONE',  ( -30.29350689640809335, 120.5696653505793705, -27.99999999999999645 ) ) ;
#7533=DIRECTION ( 'NONE',  ( 0.000000000000000000, 0.000000000000000000, -1.000000000000000000 ) ) ;
#7540=EDGE_CURVE ( 'NONE', #1359, #8958, #1405, .T. ) ;
#7553=ORIENTED_EDGE ( 'NONE', *, *, #5872, .T. ) ;
#7558=DIRECTION ( 'NONE',  ( 0.000000000000000000, 0.000000000000000000, -1.000000000000000000 ) ) ;
#7567=PLANE ( 'NONE',  #1981 ) ;
#7568=AXIS2_PLACEMENT_3D ( 'NONE', #885, #6664, #3327 ) ;
#7570=CARTESIAN_POINT ( 'NONE',  ( -30.29350689640809335, 2.445795361565304815E-15, -20.00000000000002132 ) ) ;
#7573=AXIS2_PLACEMENT_3D ( 'NONE', #1315, #8730, #3058 ) ;
#7574=DIRECTION ( 'NONE',  ( 0.000000000000000000, 0.000000000000000000, 1.000000000000000000 ) ) ;
#7575=PLANE ( 'NONE',  #8039 ) ;
#7576=CARTESIAN_POINT ( 'NONE',  ( -2.293506896408097795, 126.8146633489777599, 25.00000000000000355 ) ) ;
#7577=EDGE_CURVE ( 'NONE', #5461, #2007, #5622, .T. ) ;
#7598=DIRECTION ( 'NONE',  ( 0.000000000000000000, -1.000000000000000000, 1.222897680782651471E-16 ) ) ;
#7619=ORIENTED_EDGE ( 'NONE', *, *, #1772, .T. ) ;
#7623=ORIENTED_EDGE ( 'NONE', *, *, #9691, .T. ) ;
#7631=ORIENTED_EDGE ( 'NONE', *, *, #7513, .F. ) ;
#7633=ADVANCED_FACE ( 'NONE', ( #5670 ), #3237, .F. ) ;
#7641=ORIENTED_EDGE ( 'NONE', *, *, #2503, .F. ) ;
#7645=CARTESIAN_POINT ( 'NONE',  ( -30.29350689640809335, 120.5696653505793705, -24.00000000000000711 ) ) ;
#7654=LINE ( 'NONE', #6061, #6409 ) ;
#7658=EDGE_CURVE ( 'NONE', #1931, #941, #6469, .T. ) ;
#7660=DIRECTION ( 'NONE',  ( -1.000000000000000000, 0.000000000000000000, 0.000000000000000000 ) ) ;
#7663=ORIENTED_EDGE ( 'NONE', *, *, #3225, .F. ) ;
#7665=VECTOR ( 'NONE', #8912, 1000.000000000000000 ) ;
#7671=LINE ( 'NONE', #7570, #6701 ) ;
#7672=EDGE_CURVE ( 'NONE', #6356, #3441, #9871, .T. ) ;
#7677=LINE ( 'NONE', #2743, #1247 ) ;
#7697=ORIENTED_EDGE ( 'NONE', *, *, #8314, .T. ) ;
#7705=CARTESIAN_POINT ( 'NONE',  ( -7.293506896408097795, 72.08684478514408056, -28.00000000000001421 ) ) ;
#7715=CARTESIAN_POINT ( 'NONE',  ( -2.293506896408097795, 120.5696653505793705, -28.00000000000000355 ) ) ;
#7719=EDGE_CURVE ( 'NONE', #1403, #7054, #5772, .T. ) ;
#7726=LINE ( 'NONE', #4394, #7824 ) ;
#7736=VECTOR ( 'NONE', #2529, 1000.000000000000000 ) ;
#7737=EDGE_CURVE ( 'NONE', #6362, #2500, #66, .T. ) ;
#7744=LINE ( 'NONE', #3720, #8250 ) ;
#7751=AXIS2_PLACEMENT_3D ( 'NONE', #6579, #7473, #848 ) ;
#7756=CARTESIAN_POINT ( 'NONE',  ( -30.29350689640809335, 80.56966535057935630, -28.00000000000000355 ) ) ;
#7758=CARTESIAN_POINT ( 'NONE',  ( -30.29350689640809335, 120.5696653505793705, -20.00000000000000711 ) ) ;
#7759=VECTOR ( 'NONE', #5401, 1000.000000000000000 ) ;
#7765=EDGE_CURVE ( 'NONE', #1117, #716, #8853, .T. ) ;
#7766=CARTESIAN_POINT ( 'NONE',  ( -30.29350689640809335, 140.5696653505793563, -20.00000000000000355 ) ) ;
#7767=CIRCLE ( 'NONE', #9815, 3.999999999999993339 ) ;
#7769=CARTESIAN_POINT ( 'NONE',  ( -30.29350689640809335, 112.5696653505793705, 20.00000000000000711 ) ) ;
#7781=DIRECTION ( 'NONE',  ( 1.000000000000000000, 0.000000000000000000, 0.000000000000000000 ) ) ;
#7782=DIRECTION ( 'NONE',  ( 1.000000000000000000, 0.000000000000000000, 0.000000000000000000 ) ) ;
#7788=DIRECTION ( 'NONE',  ( 0.000000000000000000, -1.000000000000000000, -1.431206729101514631E-16 ) ) ;
#7794=ORIENTED_EDGE ( 'NONE', *, *, #7806, .T. ) ;
#7806=EDGE_CURVE ( 'NONE', #1913, #1439, #7174, .T. ) ;
#7812=LINE ( 'NONE', #10152, #1340 ) ;
#7824=VECTOR ( 'NONE', #2791, 1000.000000000000114 ) ;
#7841=VECTOR ( 'NONE', #10345, 1000.000000000000000 ) ;
#7849=AXIS2_PLACEMENT_3D ( 'NONE', #4396, #1948, #7574 ) ;
#7856=DIRECTION ( 'NONE',  ( 1.000000000000000000, -0.000000000000000000, -0.000000000000000000 ) ) ;
#7857=AXIS2_PLACEMENT_3D ( 'NONE', #4424, #7660, #5117 ) ;
#7858=LINE ( 'NONE', #657, #452 ) ;
#7862=EDGE_LOOP ( 'NONE', ( #9882, #10162, #1537, #2412 ) ) ;
#7863=CARTESIAN_POINT ( 'NONE',  ( -2.293506896408097795, 120.5696653505793705, 20.00000000000000711 ) ) ;
#7866=EDGE_CURVE ( 'NONE', #10322, #7089, #10027, .T. ) ;
#7875=CYLINDRICAL_SURFACE ( 'NONE', #1734, 4.000000000000000000 ) ;
#7880=DIRECTION ( 'NONE',  ( 0.000000000000000000, 0.000000000000000000, 1.000000000000000000 ) ) ;
#7883=EDGE_LOOP ( 'NONE', ( #7631, #6260, #3052, #3357 ) ) ;
#7891=CYLINDRICAL_SURFACE ( 'NONE', #6314, 3.999999999999989786 ) ;
#7896=AXIS2_PLACEMENT_3D ( 'NONE', #10196, #1971, #2927 ) ;
#7903=PLANE ( 'NONE',  #2116 ) ;
#7911=ORIENTED_EDGE ( 'NONE', *, *, #731, .T. ) ;
#7912=FACE_OUTER_BOUND ( 'NONE', #9391, .T. ) ;
#7915=DIRECTION ( 'NONE',  ( -1.000000000000000000, 0.000000000000000000, 0.000000000000000000 ) ) ;
#7917=VECTOR ( 'NONE', #9409, 1000.000000000000000 ) ;
#7929=FACE_OUTER_BOUND ( 'NONE', #6262, .T. ) ;
#7938=CARTESIAN_POINT ( 'NONE',  ( -30.29350689640809335, 55.56966535057937051, 0.000000000000000000 ) ) ;
#7943=CARTESIAN_POINT ( 'NONE',  ( -30.29350689640809335, 80.56966535057935630, -20.00000000000000711 ) ) ;
#7947=ORIENTED_EDGE ( 'NONE', *, *, #4771, .F. ) ;
#7948=DIRECTION ( 'NONE',  ( 0.000000000000000000, 0.000000000000000000, 1.000000000000000000 ) ) ;
#7951=DIRECTION ( 'NONE',  ( 1.000000000000000000, -0.000000000000000000, -0.000000000000000000 ) ) ;
#7955=FACE_OUTER_BOUND ( 'NONE', #9820, .T. ) ;
#7959=VERTEX_POINT ( 'NONE', #4457 ) ;
#7960=ORIENTED_EDGE ( 'NONE', *, *, #4501, .F. ) ;
#7965=CARTESIAN_POINT ( 'NONE',  ( -2.293506896408097795, 150.5696653505793563, 0.000000000000000000 ) ) ;
#7966=ORIENTED_EDGE ( 'NONE', *, *, #8084, .T. ) ;
#7967=DIRECTION ( 'NONE',  ( -1.000000000000000000, 0.000000000000000000, 0.000000000000000000 ) ) ;
#7976=AXIS2_PLACEMENT_3D ( 'NONE', #5996, #1234, #4467 ) ;
#7979=ORIENTED_EDGE ( 'NONE', *, *, #9637, .T. ) ;
#7989=VECTOR ( 'NONE', #3518, 1000.000000000000000 ) ;
#7990=ORIENTED_EDGE ( 'NONE', *, *, #1669, .T. ) ;
#7991=CARTESIAN_POINT ( 'NONE',  ( -7.293506896408097795, 0.000000000000000000, 0.000000000000000000 ) ) ;
#7994=EDGE_CURVE ( 'NONE', #1439, #4025, #3124, .T. ) ;
#7995=EDGE_LOOP ( 'NONE', ( #3912, #6914 ) ) ;
#8011=VECTOR ( 'NONE', #946, 1000.000000000000114 ) ;
#8024=DIRECTION ( 'NONE',  ( 0.000000000000000000, 0.000000000000000000, -1.000000000000000000 ) ) ;
#8031=CYLINDRICAL_SURFACE ( 'NONE', #8754, 7.500000000000000000 ) ;
#8036=DIRECTION ( 'NONE',  ( 0.000000000000000000, 0.000000000000000000, -1.000000000000000000 ) ) ;
#8038=EDGE_LOOP ( 'NONE', ( #2613, #6952 ) ) ;
#8039=AXIS2_PLACEMENT_3D ( 'NONE', #4548, #10124, #2851 ) ;
#8040=CARTESIAN_POINT ( 'NONE',  ( -16.29350689640809691, 37.08684478514406635, 7.500000000000000000 ) ) ;
#8044=DIRECTION ( 'NONE',  ( 1.000000000000000000, -0.000000000000000000, -0.000000000000000000 ) ) ;
#8054=VERTEX_POINT ( 'NONE', #3025 ) ;
#8057=DIRECTION ( 'NONE',  ( 0.000000000000000000, -1.222897680782651471E-16, 1.000000000000000000 ) ) ;
#8062=DIRECTION ( 'NONE',  ( 0.000000000000000000, -1.000000000000000000, 1.222897680782651224E-16 ) ) ;
#8068=AXIS2_PLACEMENT_3D ( 'NONE', #7991, #1682, #7948 ) ;
#8071=DIRECTION ( 'NONE',  ( 0.000000000000000000, 0.000000000000000000, 1.000000000000000000 ) ) ;
#8080=AXIS2_PLACEMENT_3D ( 'NONE', #8966, #5139, #6736 ) ;
#8081=EDGE_LOOP ( 'NONE', ( #9997, #3004, #2844, #8451, #2816 ) ) ;
#8084=EDGE_CURVE ( 'NONE', #6283, #2948, #4624, .T. ) ;
#8085=ORIENTED_EDGE ( 'NONE', *, *, #4463, .T. ) ;
#8087=DIRECTION ( 'NONE',  ( -1.000000000000000000, 0.000000000000000000, 0.000000000000000000 ) ) ;
#8088=DIRECTION ( 'NONE',  ( 0.000000000000000000, -1.222897680782651471E-16, 1.000000000000000000 ) ) ;
#8093=PLANE ( 'NONE',  #8068 ) ;
#8096=CARTESIAN_POINT ( 'NONE',  ( -24.29350689640808625, 140.5696653505793563, 20.00000000000002132 ) ) ;
#8102=CIRCLE ( 'NONE', #8611, 4.000000000000000000 ) ;
#8105=ORIENTED_EDGE ( 'NONE', *, *, #7032, .F. ) ;
#8110=DIRECTION ( 'NONE',  ( 0.000000000000000000, 0.000000000000000000, 1.000000000000000000 ) ) ;
#8112=DIRECTION ( 'NONE',  ( 0.000000000000000000, 0.000000000000000000, 1.000000000000000000 ) ) ;
#8122=DIRECTION ( 'NONE',  ( 0.000000000000000000, 0.000000000000000000, -1.000000000000000000 ) ) ;
#8124=CARTESIAN_POINT ( 'NONE',  ( -30.29350689640809335, 2.445795361565304815E-15, -20.00000000000002132 ) ) ;
#8133=EDGE_CURVE ( 'NONE', #9263, #1359, #8309, .T. ) ;
#8134=CARTESIAN_POINT ( 'NONE',  ( -30.29350689640809335, 120.5696653505793705, -20.00000000000000711 ) ) ;
#8135=AXIS2_PLACEMENT_3D ( 'NONE', #8471, #10067, #2795 ) ;
#8151=APPLICATION_CONTEXT ( 'automotive_design' ) ;
#8158=CONICAL_SURFACE ( 'NONE', #6463, 4.025000000000000355, 0.7853981633973787790 ) ;
#8164=DIRECTION ( 'NONE',  ( 1.000000000000000000, -0.000000000000000000, -0.000000000000000000 ) ) ;
#8166=CARTESIAN_POINT ( 'NONE',  ( -2.293506896408097795, 120.5696653505793705, 24.00000000000000711 ) ) ;
#8171=EDGE_CURVE ( 'NONE', #9480, #10023, #7518, .T. ) ;
#8188=ORIENTED_EDGE ( 'NONE', *, *, #302, .T. ) ;
#8191=AXIS2_PLACEMENT_3D ( 'NONE', #41, #8087, #9743 ) ;
#8193=CARTESIAN_POINT ( 'NONE',  ( -7.293506896408097795, 128.5696653505793847, 20.00000000000000711 ) ) ;
#8198=EDGE_CURVE ( 'NONE', #8054, #4361, #1637, .T. ) ;
#8207=DIRECTION ( 'NONE',  ( 0.000000000000000000, 0.000000000000000000, 1.000000000000000000 ) ) ;
#8208=DIRECTION ( 'NONE',  ( 1.000000000000000000, 0.000000000000000000, 0.000000000000000000 ) ) ;
#8216=DIRECTION ( 'NONE',  ( -1.000000000000000000, 0.000000000000000000, 0.000000000000000000 ) ) ;
#8218=CIRCLE ( 'NONE', #2638, 7.999999999999996447 ) ;
#8229=CARTESIAN_POINT ( 'NONE',  ( -20.29350689640809691, 140.5696653505793563, -20.00000000000000711 ) ) ;
#8230=CYLINDRICAL_SURFACE ( 'NONE', #376, 4.000000000000000000 ) ;
#8231=CIRCLE ( 'NONE', #5856, 7.999999999999996447 ) ;
#8236=FACE_BOUND ( 'NONE', #5377, .T. ) ;
#8237=ORIENTED_EDGE ( 'NONE', *, *, #9537, .T. ) ;
#8240=ORIENTED_EDGE ( 'NONE', *, *, #8331, .T. ) ;
#8244=VERTEX_POINT ( 'NONE', #5659 ) ;
#8250=VECTOR ( 'NONE', #10184, 1000.000000000000000 ) ;
#8256=ORIENTED_EDGE ( 'NONE', *, *, #9951, .F. ) ;
#8277=DIRECTION ( 'NONE',  ( 0.000000000000000000, 0.000000000000000000, 1.000000000000000000 ) ) ;
#8280=( NAMED_UNIT ( * ) SI_UNIT ( $, .STERADIAN. ) SOLID_ANGLE_UNIT ( ) );
#8281=ORIENTED_EDGE ( 'NONE', *, *, #4463, .F. ) ;
#8298=DIRECTION ( 'NONE',  ( 1.000000000000000000, -0.000000000000000000, -0.000000000000000000 ) ) ;
#8305=ORIENTED_EDGE ( 'NONE', *, *, #10263, .F. ) ;
#8306=CARTESIAN_POINT ( 'NONE',  ( -2.293506896408097795, 80.56966535057935630, -24.00000000000000711 ) ) ;
#8309=LINE ( 'NONE', #4284, #5979 ) ;
#8314=EDGE_CURVE ( 'NONE', #5783, #3403, #7677, .T. ) ;
#8321=AXIS2_PLACEMENT_3D ( 'NONE', #1793, #9810, #1686 ) ;
#8324=DIRECTION ( 'NONE',  ( 0.000000000000000000, 0.000000000000000000, 1.000000000000000000 ) ) ;
#8331=EDGE_CURVE ( 'NONE', #6663, #4985, #2107, .T. ) ;
#8343=ORIENTED_EDGE ( 'NONE', *, *, #3146, .T. ) ;
#8350=DIRECTION ( 'NONE',  ( -1.000000000000000000, -0.000000000000000000, -0.000000000000000000 ) ) ;
#8359=ORIENTED_EDGE ( 'NONE', *, *, #3787, .F. ) ;
#8360=DIRECTION ( 'NONE',  ( -0.000000000000000000, -0.000000000000000000, 1.000000000000000000 ) ) ;
#8361=FACE_OUTER_BOUND ( 'NONE', #2541, .T. ) ;
#8371=CARTESIAN_POINT ( 'NONE',  ( -20.29350689640809691, 140.5696653505793563, 20.00000000000002132 ) ) ;
#8382=EDGE_LOOP ( 'NONE', ( #9066, #1167, #10113, #5038 ) ) ;
#8389=EDGE_CURVE ( 'NONE', #1931, #9083, #6328, .T. ) ;
#8390=EDGE_CURVE ( 'NONE', #6365, #1352, #734, .T. ) ;
#8404=DIRECTION ( 'NONE',  ( 1.000000000000000000, -0.000000000000000000, -0.000000000000000000 ) ) ;
#8409=VECTOR ( 'NONE', #7533, 1000.000000000000000 ) ;
#8427=DIRECTION ( 'NONE',  ( -1.000000000000000000, -0.000000000000000000, -0.000000000000000000 ) ) ;
#8451=ORIENTED_EDGE ( 'NONE', *, *, #6630, .F. ) ;
#8452=VECTOR ( 'NONE', #1894, 1000.000000000000000 ) ;
#8462=ADVANCED_FACE ( 'NONE', ( #5551 ), #5595, .T. ) ;
#8468=DIRECTION ( 'NONE',  ( 0.000000000000000000, -1.000000000000000000, 0.000000000000000000 ) ) ;
#8471=CARTESIAN_POINT ( 'NONE',  ( -7.293506896408097795, 120.5696653505793705, -20.00000000000000711 ) ) ;
#8476=CARTESIAN_POINT ( 'NONE',  ( -30.29350689640809335, 120.5696653505793705, -20.00000000000000711 ) ) ;
#8481=VECTOR ( 'NONE', #6672, 1000.000000000000000 ) ;
#8485=CIRCLE ( 'NONE', #4761, 7.999999999999996447 ) ;
#8497=VECTOR ( 'NONE', #8427, 1000.000000000000000 ) ;
#8501=VECTOR ( 'NONE', #2444, 1000.000000000000000 ) ;
#8517=ORIENTED_EDGE ( 'NONE', *, *, #8653, .F. ) ;
#8529=ORIENTED_EDGE ( 'NONE', *, *, #5599, .F. ) ;
#8549=DIRECTION ( 'NONE',  ( -0.000000000000000000, -0.000000000000000000, 1.000000000000000000 ) ) ;
#8554=CARTESIAN_POINT ( 'NONE',  ( -7.293506896408097795, 120.5696653505793705, -28.00000000000000355 ) ) ;
#8560=ORIENTED_EDGE ( 'NONE', *, *, #3760, .T. ) ;
#8562=ORIENTED_EDGE ( 'NONE', *, *, #7540, .F. ) ;
#8586=CARTESIAN_POINT ( 'NONE',  ( 0.000000000000000000, 0.000000000000000000, 0.000000000000000000 ) ) ;
#8591=FACE_BOUND ( 'NONE', #781, .T. ) ;
#8595=VECTOR ( 'NONE', #4098, 1000.000000000000000 ) ;
#8601=DIRECTION ( 'NONE',  ( 1.000000000000000000, 0.000000000000000000, 0.000000000000000000 ) ) ;
#8611=AXIS2_PLACEMENT_3D ( 'NONE', #5777, #9721, #911 ) ;
#8624=ORIENTED_EDGE ( 'NONE', *, *, #3225, .T. ) ;
#8633=VERTEX_POINT ( 'NONE', #8193 ) ;
#8634=LINE ( 'NONE', #7001, #1161 ) ;
#8635=CARTESIAN_POINT ( 'NONE',  ( -16.29350689640810756, 140.5696653505793563, 20.00000000000002132 ) ) ;
#8650=FACE_OUTER_BOUND ( 'NONE', #7862, .T. ) ;
#8651=LINE ( 'NONE', #3782, #6472 ) ;
#8652=DIRECTION ( 'NONE',  ( 0.000000000000000000, 0.000000000000000000, -1.000000000000000000 ) ) ;
#8653=EDGE_CURVE ( 'NONE', #9336, #9263, #582, .T. ) ;
#8660=VECTOR ( 'NONE', #9657, 1000.000000000000000 ) ;
#8662=AXIS2_PLACEMENT_3D ( 'NONE', #4676, #6416, #4820 ) ;
#8663=CARTESIAN_POINT ( 'NONE',  ( -20.29350689640809691, 140.5696653505793563, 10.98204862120179826 ) ) ;
#8670=DIRECTION ( 'NONE',  ( 1.000000000000000000, -0.000000000000000000, -0.000000000000000000 ) ) ;
#8679=AXIS2_PLACEMENT_3D ( 'NONE', #4623, #2027, #5254 ) ;
#8689=FACE_OUTER_BOUND ( 'NONE', #3107, .T. ) ;
#8691=CARTESIAN_POINT ( 'NONE',  ( -7.293506896408097795, 4.007378841484243628E-15, 28.00000000000002132 ) ) ;
#8693=ORIENTED_EDGE ( 'NONE', *, *, #6662, .F. ) ;
#8697=EDGE_LOOP ( 'NONE', ( #10060, #5316, #4923, #9032 ) ) ;
#8704=PLANE ( 'NONE',  #8913 ) ;
#8705=DIRECTION ( 'NONE',  ( 0.000000000000000000, 0.000000000000000000, -1.000000000000000000 ) ) ;
#8706=CYLINDRICAL_SURFACE ( 'NONE', #4001, 7.999999999999989342 ) ;
#8721=FACE_OUTER_BOUND ( 'NONE', #3316, .T. ) ;
#8724=DIRECTION ( 'NONE',  ( 0.000000000000000000, 0.000000000000000000, 1.000000000000000000 ) ) ;
#8728=DIRECTION ( 'NONE',  ( 0.000000000000000000, 0.000000000000000000, -1.000000000000000000 ) ) ;
#8730=DIRECTION ( 'NONE',  ( 1.000000000000000000, -0.000000000000000000, -0.000000000000000000 ) ) ;
#8733=AXIS2_PLACEMENT_3D ( 'NONE', #10428, #2103, #1419 ) ;
#8744=AXIS2_PLACEMENT_3D ( 'NONE', #6594, #10470, #9031 ) ;
#8750=ADVANCED_FACE ( 'NONE', ( #1193 ), #353, .F. ) ;
#8752=ORIENTED_EDGE ( 'NONE', *, *, #2845, .T. ) ;
#8754=AXIS2_PLACEMENT_3D ( 'NONE', #931, #4165, #7400 ) ;
#8757=CARTESIAN_POINT ( 'NONE',  ( -30.29350689640809335, 37.08684478514406635, -15.00000000000000355 ) ) ;
#8759=DIRECTION ( 'NONE',  ( 0.000000000000000000, 0.000000000000000000, 1.000000000000000000 ) ) ;
#8766=AXIS2_PLACEMENT_3D ( 'NONE', #8229, #8923, #6534 ) ;
#8767=VERTEX_POINT ( 'NONE', #6116 ) ;
#8775=EDGE_CURVE ( 'NONE', #2946, #3592, #9898, .T. ) ;
#8779=ORIENTED_EDGE ( 'NONE', *, *, #1987, .F. ) ;
#8780=VECTOR ( 'NONE', #942, 1000.000000000000000 ) ;
#8785=CARTESIAN_POINT ( 'NONE',  ( -7.293506896408097795, 150.5696653505793563, 20.00000000000000355 ) ) ;
#8789=CARTESIAN_POINT ( 'NONE',  ( -2.293506896408097795, 150.5696653505793563, 0.000000000000000000 ) ) ;
#8791=CIRCLE ( 'NONE', #5059, 4.000000000000000000 ) ;
#8812=ORIENTED_EDGE ( 'NONE', *, *, #1786, .T. ) ;
#8815=PRODUCT ( 'Metal Mounting Block', 'Metal Mounting Block', '', ( #8932 ) ) ;
#8821=CARTESIAN_POINT ( 'NONE',  ( -30.29350689640809335, 120.5696653505793705, 20.00000000000000711 ) ) ;
#8823=CARTESIAN_POINT ( 'NONE',  ( -30.29350689640809335, 50.54838324668256888, -20.00000000000001776 ) ) ;
#8825=AXIS2_PLACEMENT_3D ( 'NONE', #3277, #6507, #9755 ) ;
#8828=EDGE_CURVE ( 'NONE', #2192, #8767, #3796, .T. ) ;
#8833=LINE ( 'NONE', #6242, #1546 ) ;
#8837=EDGE_LOOP ( 'NONE', ( #10463, #9009 ) ) ;
#8842=EDGE_CURVE ( 'NONE', #4081, #5556, #4478, .T. ) ;
#8847=CIRCLE ( 'NONE', #6284, 7.999999999999994671 ) ;
#8853=CIRCLE ( 'NONE', #1748, 4.000000000000000000 ) ;
#8854=ORIENTED_EDGE ( 'NONE', *, *, #317, .T. ) ;
#8862=LINE ( 'NONE', #5672, #3148 ) ;
#8863=VERTEX_POINT ( 'NONE', #6332 ) ;
#8872=CARTESIAN_POINT ( 'NONE',  ( -24.31850689640809549, 140.5696653505793563, 20.00000000000002132 ) ) ;
#8881=DIRECTION ( 'NONE',  ( 0.000000000000000000, 0.000000000000000000, 1.000000000000000000 ) ) ;
#8893=CARTESIAN_POINT ( 'NONE',  ( -7.293506896408097795, 126.8146633489777599, 25.00000000000000355 ) ) ;
#8894=DIRECTION ( 'NONE',  ( 1.000000000000000000, -0.000000000000000000, -0.000000000000000000 ) ) ;
#8900=ORIENTED_EDGE ( 'NONE', *, *, #1353, .T. ) ;
#8910=CARTESIAN_POINT ( 'NONE',  ( -2.293506896408097795, 4.007378841484243628E-15, 28.00000000000002132 ) ) ;
#8912=DIRECTION ( 'NONE',  ( 1.000000000000000000, 0.000000000000000000, 0.000000000000000000 ) ) ;
#8913=AXIS2_PLACEMENT_3D ( 'NONE', #5469, #8057, #801 ) ;
#8914=ORIENTED_EDGE ( 'NONE', *, *, #8389, .T. ) ;
#8918=CARTESIAN_POINT ( 'NONE',  ( -30.29350689640809335, 80.56966535057935630, -16.00000000000000711 ) ) ;
#8923=DIRECTION ( 'NONE',  ( 0.000000000000000000, -1.222897680782651471E-16, 1.000000000000000000 ) ) ;
#8924=AXIS2_PLACEMENT_3D ( 'NONE', #6656, #91, #3317 ) ;
#8931=AXIS2_PLACEMENT_3D ( 'NONE', #2067, #10136, #1331 ) ;
#8932=PRODUCT_CONTEXT ( 'NONE', #3352, 'mechanical' ) ;
#8935=ORIENTED_EDGE ( 'NONE', *, *, #4957, .T. ) ;
#8940=CYLINDRICAL_SURFACE ( 'NONE', #6192, 3.999999999999989786 ) ;
#8947=ORIENTED_EDGE ( 'NONE', *, *, #7513, .T. ) ;
#8951=DIRECTION ( 'NONE',  ( 1.000000000000000000, -0.000000000000000000, -0.000000000000000000 ) ) ;
#8956=ORIENTED_EDGE ( 'NONE', *, *, #5872, .F. ) ;
#8958=VERTEX_POINT ( 'NONE', #4837 ) ;
#8964=CARTESIAN_POINT ( 'NONE',  ( -30.29350689640809335, 120.5696653505793705, -16.00000000000000711 ) ) ;
#8966=CARTESIAN_POINT ( 'NONE',  ( 14.70649310359190309, 80.56966535057935630, 20.00000000000000711 ) ) ;
#8994=EDGE_CURVE ( 'NONE', #5189, #4587, #9048, .T. ) ;
#9003=CARTESIAN_POINT ( 'NONE',  ( -2.293506896408097795, 72.08684478514406635, 28.00000000000001066 ) ) ;
#9009=ORIENTED_EDGE ( 'NONE', *, *, #8390, .F. ) ;
#9010=EDGE_CURVE ( 'NONE', #596, #3403, #10241, .T. ) ;
#9021=CARTESIAN_POINT ( 'NONE',  ( -7.293506896408097795, -0.3998014571812398832, -1.076388538564875708 ) ) ;
#9031=DIRECTION ( 'NONE',  ( 0.000000000000000000, 0.000000000000000000, -1.000000000000000000 ) ) ;
#9032=ORIENTED_EDGE ( 'NONE', *, *, #5653, .F. ) ;
#9048=CIRCLE ( 'NONE', #3805, 4.025000000000000355 ) ;
#9050=CARTESIAN_POINT ( 'NONE',  ( -30.29350689640809335, 2.445795361565304815E-15, 20.00000000000002132 ) ) ;
#9066=ORIENTED_EDGE ( 'NONE', *, *, #356, .T. ) ;
#9067=DIRECTION ( 'NONE',  ( 0.000000000000000000, 1.000000000000000000, 0.000000000000000000 ) ) ;
#9068=AXIS2_PLACEMENT_3D ( 'NONE', #10223, #2953, #7040 ) ;
#9072=ORIENTED_EDGE ( 'NONE', *, *, #5784, .T. ) ;
#9080=CARTESIAN_POINT ( 'NONE',  ( -30.29350689640809335, 80.56966535057935630, -28.00000000000000355 ) ) ;
#9083=VERTEX_POINT ( 'NONE', #6646 ) ;
#9098=CYLINDRICAL_SURFACE ( 'NONE', #859, 7.999999999999994671 ) ;
#9113=CIRCLE ( 'NONE', #2180, 7.999999999999996447 ) ;
#9124=LINE ( 'NONE', #2705, #3845 ) ;
#9128=ADVANCED_FACE ( 'NONE', ( #8591, #3519 ), #4560, .T. ) ;
#9140=FACE_OUTER_BOUND ( 'NONE', #3830, .T. ) ;
#9172=CARTESIAN_POINT ( 'NONE',  ( -7.293506896408098683, 145.5696653505793563, 20.00000000000000711 ) ) ;
#9174=ORIENTED_EDGE ( 'NONE', *, *, #4771, .T. ) ;
#9176=VERTEX_POINT ( 'NONE', #1871 ) ;
#9181=EDGE_CURVE ( 'NONE', #1695, #6356, #3771, .T. ) ;
#9183=PLANE ( 'NONE',  #5710 ) ;
#9203=LINE ( 'NONE', #1993, #4938 ) ;
#9214=( GEOMETRIC_REPRESENTATION_CONTEXT ( 3 ) GLOBAL_UNCERTAINTY_ASSIGNED_CONTEXT ( ( #1762 ) ) GLOBAL_UNIT_ASSIGNED_CONTEXT ( ( #9279, #1956, #4321 ) ) REPRESENTATION_CONTEXT ( 'NONE', 'WORKASPACE' ) );
#9217=FACE_OUTER_BOUND ( 'NONE', #10212, .T. ) ;
#9220=AXIS2_PLACEMENT_3D ( 'NONE', #761, #7234, #6482 ) ;
#9221=ORIENTED_EDGE ( 'NONE', *, *, #2845, .F. ) ;
#9232=ORIENTED_EDGE ( 'NONE', *, *, #4696, .F. ) ;
#9236=CARTESIAN_POINT ( 'NONE',  ( -30.29350689640809335, 2.445795361565304815E-15, -20.00000000000002132 ) ) ;
#9242=CIRCLE ( 'NONE', #2464, 3.999999999999976019 ) ;
#9244=ORIENTED_EDGE ( 'NONE', *, *, #7278, .F. ) ;
#9248=DIRECTION ( 'NONE',  ( -0.000000000000000000, -0.000000000000000000, 1.000000000000000000 ) ) ;
#9258=ORIENTED_EDGE ( 'NONE', *, *, #9817, .T. ) ;
#9263=VERTEX_POINT ( 'NONE', #740 ) ;
#9270=DIRECTION ( 'NONE',  ( 0.000000000000000000, 0.000000000000000000, -1.000000000000000000 ) ) ;
#9276=ORIENTED_EDGE ( 'NONE', *, *, #2883, .F. ) ;
#9279=( LENGTH_UNIT ( ) NAMED_UNIT ( * ) SI_UNIT ( .MILLI., .METRE. ) );
#9288=ORIENTED_EDGE ( 'NONE', *, *, #5006, .F. ) ;
#9298=ORIENTED_EDGE ( 'NONE', *, *, #1516, .F. ) ;
#9306=STYLED_ITEM('',(#10497),#3077);
#9324=CARTESIAN_POINT ( 'NONE',  ( -2.293506896408097795, 120.5696653505793705, -24.00000000000000711 ) ) ;
#9326=ADVANCED_FACE ( 'NONE', ( #10299 ), #3027, .F. ) ;
#9336=VERTEX_POINT ( 'NONE', #1691 ) ;
#9337=ORIENTED_EDGE ( 'NONE', *, *, #356, .F. ) ;
#9338=AXIS2_PLACEMENT_3D ( 'NONE', #10442, #7951, #9550 ) ;
#9355=AXIS2_PLACEMENT_3D ( 'NONE', #658, #904, #850 ) ;
#9358=DIRECTION ( 'NONE',  ( -0.000000000000000000, -1.000000000000000000, -0.000000000000000000 ) ) ;
#9391=EDGE_LOOP ( 'NONE', ( #9645, #1249, #7255, #8624, #9298, #4854, #450, #5642, #4031, #4114, #383, #1442, #8935, #5344, #1339, #6058 ) ) ;
#9400=CARTESIAN_POINT ( 'NONE',  ( -30.29350689640809335, 112.5696653505793705, -20.00000000000000711 ) ) ;
#9402=LINE ( 'NONE', #3841, #3235 ) ;
#9409=DIRECTION ( 'NONE',  ( 0.7071067811864983899, 0.000000000000000000, 0.7071067811865966446 ) ) ;
#9419=CARTESIAN_POINT ( 'NONE',  ( -7.293506896408097795, 2.445795361565304815E-15, -20.00000000000002132 ) ) ;
#9453=DIRECTION ( 'NONE',  ( 0.000000000000000000, 0.000000000000000000, 1.000000000000000000 ) ) ;
#9462=VERTEX_POINT ( 'NONE', #1744 ) ;
#9472=EDGE_CURVE ( 'NONE', #5429, #5925, #270, .T. ) ;
#9474=CARTESIAN_POINT ( 'NONE',  ( -16.29350689640810756, 140.5696653505793563, -20.00000000000000711 ) ) ;
#9480=VERTEX_POINT ( 'NONE', #3551 ) ;
#9488=VERTEX_POINT ( 'NONE', #7576 ) ;
#9520=FACE_OUTER_BOUND ( 'NONE', #7503, .T. ) ;
#9522=LINE ( 'NONE', #7766, #1485 ) ;
#9530=VECTOR ( 'NONE', #10119, 1000.000000000000000 ) ;
#9532=CIRCLE ( 'NONE', #10200, 10.00000000000000888 ) ;
#9537=EDGE_CURVE ( 'NONE', #5925, #6085, #1706, .T. ) ;
#9544=CARTESIAN_POINT ( 'NONE',  ( -30.29350689640809335, 80.56966535057935630, -20.00000000000000711 ) ) ;
#9546=DIRECTION ( 'NONE',  ( -0.000000000000000000, -0.000000000000000000, -1.000000000000000000 ) ) ;
#9547=VECTOR ( 'NONE', #1276, 1000.000000000000000 ) ;
#9550=DIRECTION ( 'NONE',  ( 0.000000000000000000, 0.000000000000000000, -1.000000000000000000 ) ) ;
#9576=DIRECTION ( 'NONE',  ( -1.000000000000000000, 0.000000000000000000, 0.000000000000000000 ) ) ;
#9590=LINE ( 'NONE', #4702, #5679 ) ;
#9591=FACE_OUTER_BOUND ( 'NONE', #1268, .T. ) ;
#9593=DIRECTION ( 'NONE',  ( 1.000000000000000000, -0.000000000000000000, -0.000000000000000000 ) ) ;
#9594=VECTOR ( 'NONE', #2509, 1000.000000000000000 ) ;
#9601=CARTESIAN_POINT ( 'NONE',  ( -7.293506896408097795, 72.08684478514408056, -28.00000000000001421 ) ) ;
#9611=ORIENTED_EDGE ( 'NONE', *, *, #2121, .T. ) ;
#9615=EDGE_CURVE ( 'NONE', #1282, #6490, #8833, .T. ) ;
#9619=CLOSED_SHELL ( 'NONE', ( #3870, #9326, #4534, #4757, #3852, #6967, #4564, #8750, #2737, #5421, #6159, #8462, #3414, #9722, #6819, #3596, #545, #489, #9128, #4502, #3523, #1845, #1654, #2235, #5084, #2292, #1468, #6189, #9963, #7633, #3474, #4164, #5949, #10073, #5057, #89, #9737, #5683, #9903, #6855, #2109, #4428, #4876, #10203, #4488, #676, #1773, #7095, #5820, #3527, #1407, #2535 ) ) ;
#9629=EDGE_LOOP ( 'NONE', ( #1196, #1418, #8900, #4505 ) ) ;
#9630=PLANE ( 'NONE',  #6725 ) ;
#9637=EDGE_CURVE ( 'NONE', #5715, #6490, #6396, .T. ) ;
#9638=EDGE_LOOP ( 'NONE', ( #2257, #5071, #875, #7697 ) ) ;
#9645=ORIENTED_EDGE ( 'NONE', *, *, #3673, .T. ) ;
#9657=DIRECTION ( 'NONE',  ( -0.000000000000000000, -0.000000000000000000, 1.000000000000000000 ) ) ;
#9688=FACE_BOUND ( 'NONE', #8038, .T. ) ;
#9691=EDGE_CURVE ( 'NONE', #5461, #4081, #777, .T. ) ;
#9698=ORIENTED_EDGE ( 'NONE', *, *, #1199, .F. ) ;
#9708=EDGE_CURVE ( 'NONE', #716, #5577, #4018, .T. ) ;
#9717=AXIS2_PLACEMENT_3D ( 'NONE', #2902, #4547, #7781 ) ;
#9720=ORIENTED_EDGE ( 'NONE', *, *, #9708, .T. ) ;
#9721=DIRECTION ( 'NONE',  ( -1.000000000000000000, 0.000000000000000000, 0.000000000000000000 ) ) ;
#9722=ADVANCED_FACE ( 'NONE', ( #5063 ), #9098, .T. ) ;
#9732=CARTESIAN_POINT ( 'NONE',  ( -30.29350689640809335, 120.5696653505793705, -16.00000000000000711 ) ) ;
#9737=ADVANCED_FACE ( 'NONE', ( #152 ), #3378, .F. ) ;
#9739=VECTOR ( 'NONE', #10242, 1000.000000000000000 ) ;
#9743=DIRECTION ( 'NONE',  ( 0.000000000000000000, 0.000000000000000000, 1.000000000000000000 ) ) ;
#9746=CARTESIAN_POINT ( 'NONE',  ( -30.29350689640809335, 120.5696653505793705, 20.00000000000000711 ) ) ;
#9748=ORIENTED_EDGE ( 'NONE', *, *, #5173, .F. ) ;
#9755=DIRECTION ( 'NONE',  ( 0.000000000000000000, 0.000000000000000000, -1.000000000000000000 ) ) ;
#9774=AXIS2_PLACEMENT_3D ( 'NONE', #5575, #7915, #8759 ) ;
#9786=CARTESIAN_POINT ( 'NONE',  ( -16.29350689640809691, -19.43033464942062238, 7.500000000000000000 ) ) ;
#9801=DIRECTION ( 'NONE',  ( 0.000000000000000000, 1.460512169908342690E-16, -1.000000000000000000 ) ) ;
#9806=CARTESIAN_POINT ( 'NONE',  ( -20.29350689640809691, 140.5696653505793563, -10.98204862120179648 ) ) ;
#9810=DIRECTION ( 'NONE',  ( 0.000000000000000000, -1.460512169908342690E-16, -1.000000000000000000 ) ) ;
#9815=AXIS2_PLACEMENT_3D ( 'NONE', #3631, #9248, #504 ) ;
#9816=VERTEX_POINT ( 'NONE', #4954 ) ;
#9817=EDGE_CURVE ( 'NONE', #2923, #9462, #6498, .T. ) ;
#9820=EDGE_LOOP ( 'NONE', ( #1071, #9848, #6089, #4246, #1069 ) ) ;
#9836=CARTESIAN_POINT ( 'NONE',  ( -30.29350689640809335, 80.56966535057935630, -20.00000000000000711 ) ) ;
#9838=DIRECTION ( 'NONE',  ( 0.000000000000000000, -1.000000000000000000, -1.222897680782651224E-16 ) ) ;
#9848=ORIENTED_EDGE ( 'NONE', *, *, #5909, .F. ) ;
#9851=VECTOR ( 'NONE', #95, 1000.000000000000000 ) ;
#9855=CARTESIAN_POINT ( 'NONE',  ( -7.293506896408097795, 120.5696653505793705, 28.00000000000000355 ) ) ;
#9856=ORIENTED_EDGE ( 'NONE', *, *, #3900, .T. ) ;
#9857=AXIS2_PLACEMENT_3D ( 'NONE', #3334, #8894, #6564 ) ;
#9864=DIRECTION ( 'NONE',  ( 0.000000000000000000, -1.000000000000000000, 1.222897680782651224E-16 ) ) ;
#9871=CIRCLE ( 'NONE', #9355, 7.999999999999994671 ) ;
#9880=DIRECTION ( 'NONE',  ( 0.000000000000000000, 0.000000000000000000, 1.000000000000000000 ) ) ;
#9882=ORIENTED_EDGE ( 'NONE', *, *, #9964, .F. ) ;
#9895=DIRECTION ( 'NONE',  ( 0.000000000000000000, -1.000000000000000000, 1.222897680782651224E-16 ) ) ;
#9898=CIRCLE ( 'NONE', #7857, 4.000000000000000000 ) ;
#9903=ADVANCED_FACE ( 'NONE', ( #5119 ), #3637, .T. ) ;
#9905=FACE_OUTER_BOUND ( 'NONE', #4790, .T. ) ;
#9922=CIRCLE ( 'NONE', #763, 7.500000000000000000 ) ;
#9928=AXIS2_PLACEMENT_3D ( 'NONE', #6226, #2201, #667 ) ;
#9941=FACE_OUTER_BOUND ( 'NONE', #6737, .T. ) ;
#9945=LINE ( 'NONE', #3410, #7989 ) ;
#9951=EDGE_CURVE ( 'NONE', #5556, #4617, #4934, .T. ) ;
#9962=CARTESIAN_POINT ( 'NONE',  ( -7.293506896408097795, 112.5696653505793705, -20.00000000000000711 ) ) ;
#9963=ADVANCED_FACE ( 'NONE', ( #9941 ), #8230, .F. ) ;
#9964=EDGE_CURVE ( 'NONE', #9083, #9176, #5100, .T. ) ;
#9967=VECTOR ( 'NONE', #5303, 1000.000000000000000 ) ;
#9970=CARTESIAN_POINT ( 'NONE',  ( -2.293506896408097795, 55.56966535057937051, -10.98204862120179826 ) ) ;
#9971=DIRECTION ( 'NONE',  ( 1.000000000000000000, -0.000000000000000000, -0.000000000000000000 ) ) ;
#9978=ORIENTED_EDGE ( 'NONE', *, *, #7022, .T. ) ;
#9983=DIRECTION ( 'NONE',  ( 1.000000000000000000, -0.000000000000000000, -0.000000000000000000 ) ) ;
#9988=( NAMED_UNIT ( * ) PLANE_ANGLE_UNIT ( ) SI_UNIT ( $, .RADIAN. ) );
#9997=ORIENTED_EDGE ( 'NONE', *, *, #1006, .T. ) ;
#9999=ORIENTED_EDGE ( 'NONE', *, *, #1594, .T. ) ;
#10000=DIRECTION ( 'NONE',  ( 1.000000000000000000, -0.000000000000000000, -0.000000000000000000 ) ) ;
#10001=ORIENTED_EDGE ( 'NONE', *, *, #8171, .F. ) ;
#10023=VERTEX_POINT ( 'NONE', #544 ) ;
#10027=LINE ( 'NONE', #10134, #9547 ) ;
#10028=CARTESIAN_POINT ( 'NONE',  ( -7.293506896408097795, 4.007378841484243628E-15, 28.00000000000002132 ) ) ;
#10030=DIRECTION ( 'NONE',  ( -0.000000000000000000, 1.000000000000000000, -0.000000000000000000 ) ) ;
#10031=ORIENTED_EDGE ( 'NONE', *, *, #2245, .F. ) ;
#10053=DIRECTION ( 'NONE',  ( 0.000000000000000000, -1.734723475976808278E-15, 1.000000000000000000 ) ) ;
#10060=ORIENTED_EDGE ( 'NONE', *, *, #2627, .F. ) ;
#10063=CIRCLE ( 'NONE', #255, 7.500000000000000000 ) ;
#10064=LINE ( 'NONE', #6772, #832 ) ;
#10065=CARTESIAN_POINT ( 'NONE',  ( -2.293506896408097795, -0.3998014571812398832, -1.076388538564875708 ) ) ;
#10067=DIRECTION ( 'NONE',  ( 1.000000000000000000, -0.000000000000000000, -0.000000000000000000 ) ) ;
#10073=ADVANCED_FACE ( 'NONE', ( #5252 ), #2818, .F. ) ;
#10080=DIRECTION ( 'NONE',  ( 0.000000000000000000, -1.000000000000000000, 1.431206729101514631E-16 ) ) ;
#10087=EDGE_CURVE ( 'NONE', #5429, #4328, #2764, .T. ) ;
#10089=FACE_OUTER_BOUND ( 'NONE', #9638, .T. ) ;
#10109=VECTOR ( 'NONE', #4198, 1000.000000000000000 ) ;
#10111=ORIENTED_EDGE ( 'NONE', *, *, #5713, .F. ) ;
#10113=ORIENTED_EDGE ( 'NONE', *, *, #3673, .F. ) ;
#10115=ORIENTED_EDGE ( 'NONE', *, *, #1772, .F. ) ;
#10119=DIRECTION ( 'NONE',  ( 0.000000000000000000, -1.000000000000000000, -1.431206729101514631E-16 ) ) ;
#10122=VECTOR ( 'NONE', #8164, 1000.000000000000000 ) ;
#10124=DIRECTION ( 'NONE',  ( 0.000000000000000000, -1.000000000000000000, -0.000000000000000000 ) ) ;
#10127=ORIENTED_EDGE ( 'NONE', *, *, #6146, .F. ) ;
#10134=CARTESIAN_POINT ( 'NONE',  ( -30.29350689640809335, 128.5696653505793563, -20.00000000000000711 ) ) ;
#10136=DIRECTION ( 'NONE',  ( -1.000000000000000000, 0.000000000000000000, 0.000000000000000000 ) ) ;
#10137=EDGE_LOOP ( 'NONE', ( #3972, #5952, #1100, #6517 ) ) ;
#10138=ORIENTED_EDGE ( 'NONE', *, *, #6932, .F. ) ;
#10141=ORIENTED_EDGE ( 'NONE', *, *, #8171, .T. ) ;
#10150=VECTOR ( 'NONE', #9864, 1000.000000000000000 ) ;
#10151=DIRECTION ( 'NONE',  ( 1.000000000000000000, -0.000000000000000000, -0.000000000000000000 ) ) ;
#10152=CARTESIAN_POINT ( 'NONE',  ( -30.29350689640809335, 150.5696653505793563, 20.00000000000000355 ) ) ;
#10156=LINE ( 'NONE', #1354, #4852 ) ;
#10162=ORIENTED_EDGE ( 'NONE', *, *, #8389, .F. ) ;
#10164=VERTEX_POINT ( 'NONE', #7645 ) ;
#10178=CARTESIAN_POINT ( 'NONE',  ( -2.293506896408097795, 55.56966535057937051, 10.98204862120179826 ) ) ;
#10184=DIRECTION ( 'NONE',  ( 1.000000000000000000, -0.000000000000000000, -0.000000000000000000 ) ) ;
#10191=ORIENTED_EDGE ( 'NONE', *, *, #7010, .T. ) ;
#10196=CARTESIAN_POINT ( 'NONE',  ( -2.293506896408097795, 120.5696653505793705, 20.00000000000000711 ) ) ;
#10200=AXIS2_PLACEMENT_3D ( 'NONE', #1148, #4385, #6813 ) ;
#10203=ADVANCED_FACE ( 'NONE', ( #10308, #3985 ), #656, .T. ) ;
#10212=EDGE_LOOP ( 'NONE', ( #2812, #419, #7979, #3145, #7663 ) ) ;
#10217=ORIENTED_EDGE ( 'NONE', *, *, #1532, .T. ) ;
#10223=CARTESIAN_POINT ( 'NONE',  ( -30.29350689640809335, 2.445795361565304815E-15, 20.00000000000002132 ) ) ;
#10237=LINE ( 'NONE', #8635, #8660 ) ;
#10241=CIRCLE ( 'NONE', #9220, 7.999999999999996447 ) ;
#10242=DIRECTION ( 'NONE',  ( 1.000000000000000000, -0.000000000000000000, -0.000000000000000000 ) ) ;
#10250=CARTESIAN_POINT ( 'NONE',  ( -7.293506896408097795, 120.5696653505793705, 20.00000000000000711 ) ) ;
#10254=ORIENTED_EDGE ( 'NONE', *, *, #8994, .F. ) ;
#10257=LINE ( 'NONE', #2035, #467 ) ;
#10258=VECTOR ( 'NONE', #3047, 1000.000000000000000 ) ;
#10263=EDGE_CURVE ( 'NONE', #10023, #4985, #1596, .T. ) ;
#10264=VERTEX_POINT ( 'NONE', #5468 ) ;
#10265=DIRECTION ( 'NONE',  ( 1.000000000000000000, -0.000000000000000000, -0.000000000000000000 ) ) ;
#10266=VECTOR ( 'NONE', #10378, 1000.000000000000000 ) ;
#10269=ORIENTED_EDGE ( 'NONE', *, *, #2872, .F. ) ;
#10287=AXIS2_PLACEMENT_3D ( 'NONE', #9806, #4124, #5753 ) ;
#10299=FACE_OUTER_BOUND ( 'NONE', #2206, .T. ) ;
#10302=VECTOR ( 'NONE', #10080, 1000.000000000000000 ) ;
#10304=CIRCLE ( 'NONE', #3874, 4.025000000000000355 ) ;
#10308=FACE_BOUND ( 'NONE', #7470, .T. ) ;
#10312=ORIENTED_EDGE ( 'NONE', *, *, #2943, .F. ) ;
#10319=DIRECTION ( 'NONE',  ( 0.000000000000000000, 0.000000000000000000, -1.000000000000000000 ) ) ;
#10322=VERTEX_POINT ( 'NONE', #4292 ) ;
#10323=CARTESIAN_POINT ( 'NONE',  ( -30.29350689640809335, 150.5696653505793563, 0.000000000000000000 ) ) ;
#10332=CARTESIAN_POINT ( 'NONE',  ( -7.293506896408105789, 88.56966535057934209, 20.00000000000001066 ) ) ;
#10339=EDGE_CURVE ( 'NONE', #9488, #5863, #1060, .T. ) ;
#10344=CARTESIAN_POINT ( 'NONE',  ( -7.293506896408097795, 80.56966535057935630, 20.00000000000000711 ) ) ;
#10345=DIRECTION ( 'NONE',  ( 1.000000000000000000, 0.000000000000000000, 0.000000000000000000 ) ) ;
#10346=DIRECTION ( 'NONE',  ( 0.000000000000000000, 1.431206729101514631E-16, 1.000000000000000000 ) ) ;
#10352=EDGE_LOOP ( 'NONE', ( #8914, #10217 ) ) ;
#10358=ORIENTED_EDGE ( 'NONE', *, *, #2487, .T. ) ;
#10359=DIRECTION ( 'NONE',  ( 0.000000000000000000, 0.000000000000000000, 1.000000000000000000 ) ) ;
#10368=CARTESIAN_POINT ( 'NONE',  ( -2.293506896408097795, 37.08684478514406635, -15.00000000000000355 ) ) ;
#10378=DIRECTION ( 'NONE',  ( 0.000000000000000000, 0.000000000000000000, -1.000000000000000000 ) ) ;
#10379=DIRECTION ( 'NONE',  ( 1.000000000000000000, 0.000000000000000000, 0.000000000000000000 ) ) ;
#10390=CARTESIAN_POINT ( 'NONE',  ( -2.293506896408097795, 120.5696653505793705, 28.00000000000000355 ) ) ;
#10408=EDGE_CURVE ( 'NONE', #8958, #9336, #2062, .T. ) ;
#10423=CARTESIAN_POINT ( 'NONE',  ( -2.293506896408097795, 120.5696653505793705, -16.00000000000000711 ) ) ;
#10424=ORIENTED_EDGE ( 'NONE', *, *, #1380, .T. ) ;
#10428=CARTESIAN_POINT ( 'NONE',  ( -20.29350689640809691, 140.5696653505793563, 10.98204862120179826 ) ) ;
#10442=CARTESIAN_POINT ( 'NONE',  ( -30.29350689640809335, 80.56966535057935630, -20.00000000000000711 ) ) ;
#10445=DIRECTION ( 'NONE',  ( 1.000000000000000000, -0.000000000000000000, -0.000000000000000000 ) ) ;
#10463=ORIENTED_EDGE ( 'NONE', *, *, #3146, .F. ) ;
#10470=DIRECTION ( 'NONE',  ( 0.000000000000000000, -1.000000000000000000, -0.000000000000000000 ) ) ;
#10471=ORIENTED_EDGE ( 'NONE', *, *, #7483, .T. ) ;
#10473=ORIENTED_EDGE ( 'NONE', *, *, #1140, .T. ) ;
#10475=LINE ( 'NONE', #8823, #2515 ) ;
#10478=PLANE ( 'NONE',  #8321 ) ;
#10491=COLOUR_RGB('Dark Blue',0.08,0.2,0.34);
#10492=FILL_AREA_STYLE_COLOUR('',#10491);
#10493=FILL_AREA_STYLE('',(#10492));
#10494=SURFACE_STYLE_FILL_AREA(#10493);
#10495=SURFACE_SIDE_STYLE('',(#10494));
#10496=SURFACE_STYLE_USAGE(.BOTH.,#10495);
#10497=PRESENTATION_STYLE_ASSIGNMENT((#10496));
ENDSEC;
END-ISO-10303-21;
